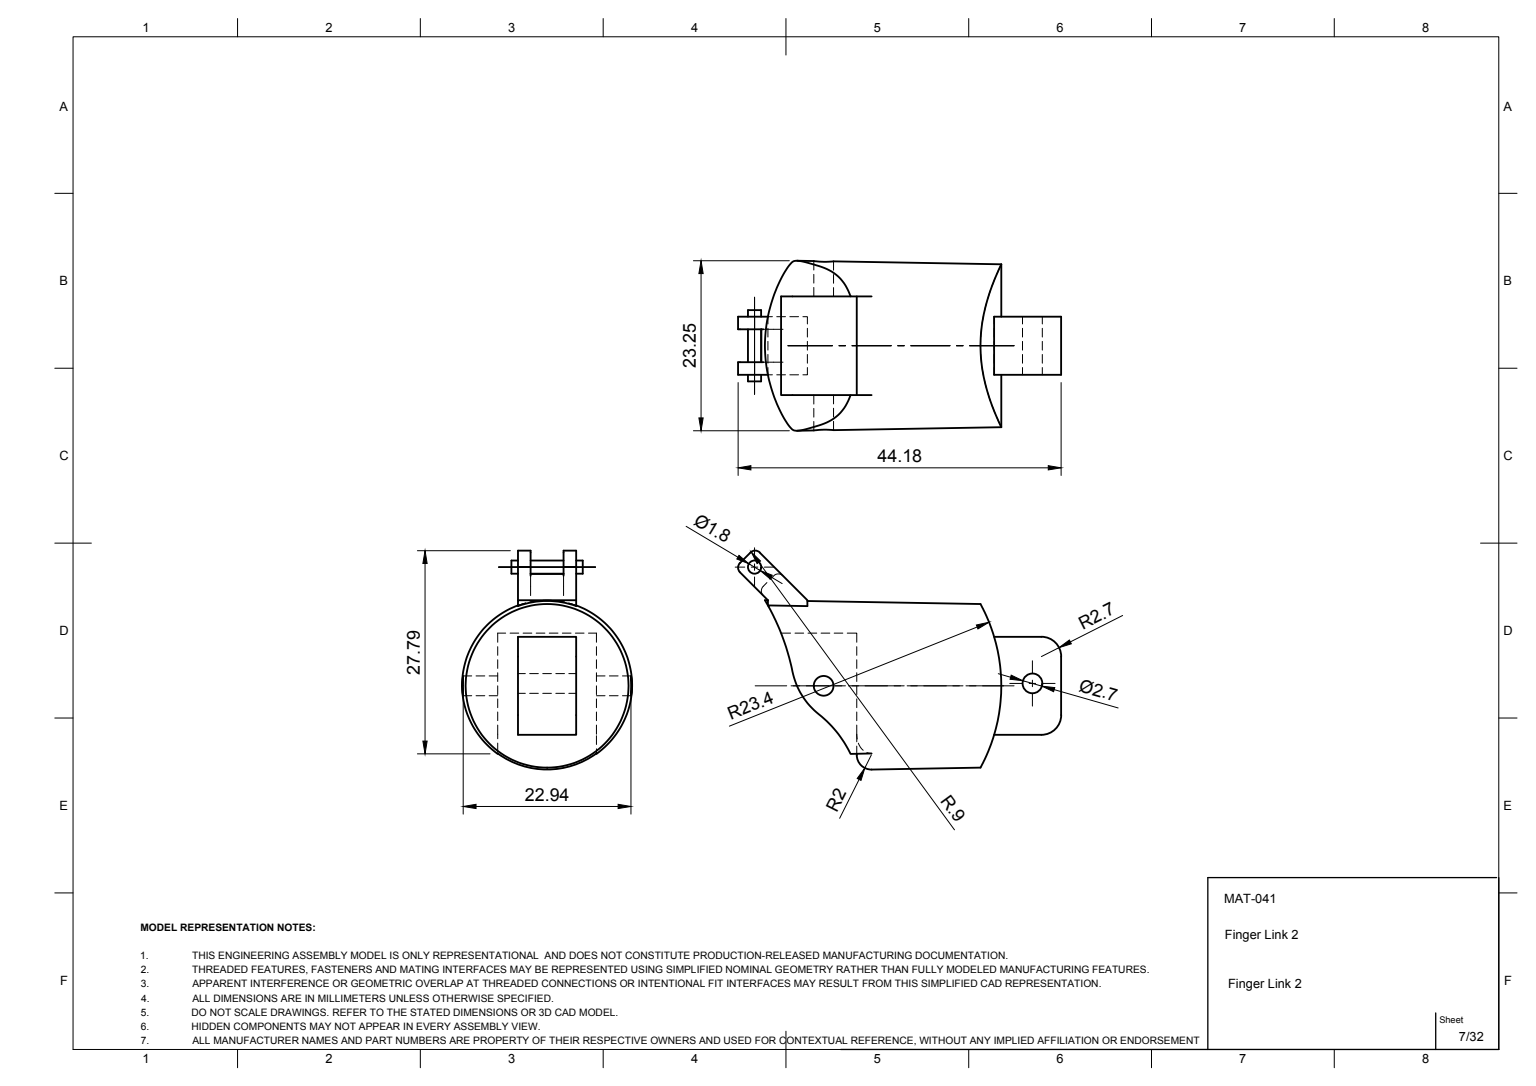
ISO-10303-21;
HEADER;
/* Generated by software containing ST-Developer
 * from STEP Tools, Inc. (www.steptools.com) 
 */

FILE_DESCRIPTION(
/* description */ ('STEP AP214'),
/* implementation_level */ '2;1');

FILE_NAME(
/* name */ 'Finger Link 2.step',
/* time_stamp */ '2026-11-14T21:57:47-08:00',
/* author */ (''),
/* organization */ (''),
/* preprocessor_version */ 'ST-DEVELOPER v20.2',
/* originating_system */ 'Autodesk Translation Framework v15.17.0.0',
/* authorisation */ '');

FILE_SCHEMA (('AUTOMOTIVE_DESIGN { 1 0 10303 214 3 1 1 }'));
ENDSEC;

DATA;
#10=MECHANICAL_DESIGN_GEOMETRIC_PRESENTATION_REPRESENTATION('',(#250),#13199);
#119=CONICAL_SURFACE('',#7291,11.7,0.0174532925199433);
#120=CONICAL_SURFACE('',#7299,11.7,0.0174532925199433);
#141=B_SPLINE_CURVE_WITH_KNOTS('',3,(#10617,#10618,#10619,#10620,#10621,
#10622,#10623,#10624,#10625,#10626,#10627,#10628,#10629,#10630,#10631,#10632,
#10633,#10634),.UNSPECIFIED.,.F.,.F.,(4,2,2,2,2,2,2,2,4),(1.0177645095144,
1.06859347183877,1.11942243416314,1.17022390747156,1.22102538077998,1.27203011389648,
1.32303484701297,1.37402558782589,1.42501632863882),.UNSPECIFIED.);
#142=B_SPLINE_CURVE_WITH_KNOTS('',3,(#10635,#10636,#10637,#10638,#10639,
#10640,#10641,#10642,#10643,#10644,#10645,#10646,#10647,#10648,#10649,#10650,
#10651,#10652,#10653),.UNSPECIFIED.,.F.,.F.,(4,2,2,2,3,2,2,2,4),(0.610512690389992,
0.661503431202914,0.712494172015835,0.763498905132329,0.814503638248823,
0.865305111557246,0.916106584865669,0.966935547190036,1.0177645095144),
 .UNSPECIFIED.);
#143=B_SPLINE_CURVE_WITH_KNOTS('',3,(#10657,#10658,#10659,#10660,#10661,
#10662,#10663,#10664,#10665,#10666,#10667,#10668,#10669,#10670,#10671,#10672,
#10673,#10674),.UNSPECIFIED.,.F.,.F.,(4,2,2,2,2,2,2,2,4),(-0.610512690389992,
-0.55952194957707,-0.508531208764149,-0.457526475647655,-0.406521742531161,
-0.355720269222738,-0.304918795914315,-0.254089833589948,-0.203260871265581),
 .UNSPECIFIED.);
#144=B_SPLINE_CURVE_WITH_KNOTS('',3,(#10678,#10679,#10680,#10681,#10682,
#10683,#10684,#10685,#10686,#10687,#10688,#10689,#10690,#10691,#10692,#10693,
#10694,#10695,#10696),.UNSPECIFIED.,.F.,.F.,(4,2,2,2,3,2,2,2,4),(-0.203260871265581,
-0.152431908941213,-0.101602946616846,-0.0508014733084231,0.,0.0510047331164938,
0.102009466232988,0.153000207045909,0.203990947858831),.UNSPECIFIED.);
#145=B_SPLINE_CURVE_WITH_KNOTS('',3,(#10702,#10703,#10704,#10705),
 .UNSPECIFIED.,.F.,.F.,(4,4),(0.0320334028505474,0.0349204253098787),
 .UNSPECIFIED.);
#146=B_SPLINE_CURVE_WITH_KNOTS('',3,(#10707,#10708,#10709,#10710,#10711,
#10712,#10713,#10714,#10715,#10716),.UNSPECIFIED.,.F.,.F.,(4,2,2,2,4),(1.8422488924149,
2.04440794331246,2.28720862023162,2.53000929715077,2.64124356821964),
 .UNSPECIFIED.);
#147=B_SPLINE_CURVE_WITH_KNOTS('',3,(#10718,#10719,#10720,#10721,#10722,
#10723,#10724,#10725,#10726,#10727),.UNSPECIFIED.,.F.,.F.,(4,2,2,2,4),(6.38658386410106,
6.48595628344589,6.66853921041904,6.85112213739218,7.0623660754825),
 .UNSPECIFIED.);
#148=B_SPLINE_CURVE_WITH_KNOTS('',3,(#10729,#10730,#10731,#10732,#10733,
#10734,#10735,#10736,#10737,#10738),.UNSPECIFIED.,.F.,.F.,(4,2,2,2,4),(3.96444278282234,
4.01597597737689,4.46288213733859,4.92120866579123,5.18441802586752),
 .UNSPECIFIED.);
#149=B_SPLINE_CURVE_WITH_KNOTS('',3,(#10740,#10741,#10742,#10743,#10744,
#10745,#10746),.UNSPECIFIED.,.F.,.F.,(4,3,4),(0.0201480402418329,0.0228906128443418,
0.0255489715004856),.UNSPECIFIED.);
#150=B_SPLINE_CURVE_WITH_KNOTS('',3,(#10752,#10753,#10754,#10755,#10756,
#10757,#10758,#10759,#10760,#10761,#10762,#10763,#10764,#10765,#10766,#10767,
#10768,#10769,#10770,#10771,#10772,#10773),.UNSPECIFIED.,.F.,.F.,(4,2,2,
2,2,2,2,2,2,2,4),(3.42549582701687,3.63995923491168,3.8544226428065,4.28334945859613,
4.71079343465883,5.13823741072153,5.56568618497645,5.99313495923137,6.42206330663255,
6.63652748033314,6.85099165403373),.UNSPECIFIED.);
#151=B_SPLINE_CURVE_WITH_KNOTS('',3,(#10774,#10775,#10776,#10777,#10778,
#10779,#10780,#10781,#10782,#10783,#10784,#10785,#10786,#10787,#10788,#10789,
#10790,#10791,#10792,#10793,#10794,#10795),.UNSPECIFIED.,.F.,.F.,(4,2,2,
2,2,2,2,2,2,2,4),(0.,0.21446417370059,0.428928347401181,0.857856694802362,
1.28530546905728,1.7127542433122,2.1401982193749,2.5676421954376,2.99656901122723,
3.21103241912205,3.42549582701687),.UNSPECIFIED.);
#152=B_SPLINE_CURVE_WITH_KNOTS('',3,(#10799,#10800,#10801,#10802,#10803,
#10804,#10805),.UNSPECIFIED.,.F.,.F.,(4,3,4),(0.0202322541917222,0.0228906128474993,
0.0256331854496299),.UNSPECIFIED.);
#153=B_SPLINE_CURVE_WITH_KNOTS('',3,(#10807,#10808,#10809,#10810,#10811,
#10812,#10813,#10814,#10815,#10816),.UNSPECIFIED.,.F.,.F.,(4,2,2,2,4),(1.95372160896285,
2.21693096903914,2.67525749749178,3.12216365745348,3.17369685200803),
 .UNSPECIFIED.);
#154=B_SPLINE_CURVE_WITH_KNOTS('',3,(#10818,#10819,#10820,#10821,#10822,
#10823,#10824,#10825,#10826,#10827),.UNSPECIFIED.,.F.,.F.,(4,2,2,2,4),(10.2613045765272,
10.4725485146175,10.6551314415907,10.8377143685638,10.9370867879086),
 .UNSPECIFIED.);
#155=B_SPLINE_CURVE_WITH_KNOTS('',3,(#10829,#10830,#10831,#10832,#10833,
#10834,#10835,#10836,#10837,#10838),.UNSPECIFIED.,.F.,.F.,(4,2,2,2,4),(4.03342707380782,
4.14466134487669,4.38746202179585,4.630262698715,4.83242174961257),
 .UNSPECIFIED.);
#156=B_SPLINE_CURVE_WITH_KNOTS('',3,(#10839,#10840,#10841,#10842),
 .UNSPECIFIED.,.F.,.F.,(4,4),(0.0108996070094278,0.0137866294584668),
 .UNSPECIFIED.);
#157=B_SPLINE_CURVE_WITH_KNOTS('',3,(#10848,#10849,#10850,#10851,#10852,
#10853,#10854,#10855,#10856,#10857),.UNSPECIFIED.,.F.,.F.,(4,2,2,2,4),(-3.96444278282234,
-3.79252289739604,-3.56906981741519,-3.34561673743433,-3.17369685200803),
 .UNSPECIFIED.);
#158=B_SPLINE_CURVE_WITH_KNOTS('',3,(#10897,#10898,#10899,#10900,#10901,
#10902,#10903,#10904,#10905,#10906,#10907,#10908,#10909),.UNSPECIFIED.,
 .F.,.F.,(4,2,2,2,3,4),(-0.346533453564935,-0.234184438198016,-0.144253134532049,
-0.0681159640541859,0.,0.00346167201765239),.UNSPECIFIED.);
#159=B_SPLINE_CURVE_WITH_KNOTS('',3,(#10914,#10915,#10916,#10917,#10918,
#10919,#10920,#10921,#10922,#10923,#10924,#10925,#10926),.UNSPECIFIED.,
 .F.,.F.,(4,3,2,2,2,4),(-0.003464253118063,0.,0.0681159640541862,0.14425313453205,
0.234184438198017,0.346533453564935),.UNSPECIFIED.);
#214=SHAPE_REPRESENTATION_RELATIONSHIP('SRR','None',#13282,#232);
#232=ADVANCED_BREP_SHAPE_REPRESENTATION('',(#268),#13178);
#250=STYLED_ITEM('',(#13409),#268);
#268=MANIFOLD_SOLID_BREP('Body1',#6845);
#301=FACE_BOUND('',#2318,.T.);
#302=FACE_BOUND('',#2319,.T.);
#303=FACE_BOUND('',#2324,.T.);
#304=FACE_BOUND('',#2327,.T.);
#305=FACE_BOUND('',#2329,.T.);
#306=FACE_BOUND('',#2333,.T.);
#307=FACE_BOUND('',#2336,.T.);
#308=FACE_BOUND('',#2342,.T.);
#309=FACE_BOUND('',#2344,.T.);
#310=FACE_BOUND('',#2355,.T.);
#311=FACE_BOUND('',#2358,.T.);
#441=PLANE('',#7298);
#442=PLANE('',#7304);
#443=PLANE('',#7306);
#444=PLANE('',#7309);
#445=PLANE('',#7312);
#446=PLANE('',#7313);
#447=PLANE('',#7314);
#448=PLANE('',#7317);
#449=PLANE('',#7318);
#450=PLANE('',#7321);
#451=PLANE('',#7322);
#452=PLANE('',#7323);
#453=PLANE('',#7324);
#454=PLANE('',#7325);
#455=PLANE('',#7330);
#456=PLANE('',#7335);
#457=PLANE('',#7336);
#458=PLANE('',#7343);
#459=PLANE('',#7344);
#460=PLANE('',#7347);
#461=PLANE('',#7348);
#462=PLANE('',#7351);
#734=LINE('',#10591,#1252);
#735=LINE('',#10597,#1253);
#736=LINE('',#10603,#1254);
#737=LINE('',#10609,#1255);
#738=LINE('',#10615,#1256);
#739=LINE('',#10676,#1257);
#740=LINE('',#10750,#1258);
#741=LINE('',#10847,#1259);
#742=LINE('',#10859,#1260);
#743=LINE('',#10862,#1261);
#744=LINE('',#10866,#1262);
#745=LINE('',#10868,#1263);
#746=LINE('',#10870,#1264);
#747=LINE('',#10871,#1265);
#748=LINE('',#10877,#1266);
#749=LINE('',#10881,#1267);
#750=LINE('',#10888,#1268);
#751=LINE('',#10890,#1269);
#752=LINE('',#10891,#1270);
#753=LINE('',#10896,#1271);
#754=LINE('',#10927,#1272);
#755=LINE('',#10931,#1273);
#756=LINE('',#10933,#1274);
#757=LINE('',#10934,#1275);
#758=LINE('',#10938,#1276);
#759=LINE('',#10942,#1277);
#760=LINE('',#10943,#1278);
#761=LINE('',#10945,#1279);
#762=LINE('',#10949,#1280);
#763=LINE('',#10950,#1281);
#764=LINE('',#10953,#1282);
#765=LINE('',#10957,#1283);
#766=LINE('',#10960,#1284);
#767=LINE('',#10962,#1285);
#768=LINE('',#10964,#1286);
#769=LINE('',#10966,#1287);
#770=LINE('',#10967,#1288);
#771=LINE('',#10971,#1289);
#772=LINE('',#10973,#1290);
#773=LINE('',#10975,#1291);
#774=LINE('',#10976,#1292);
#775=LINE('',#10977,#1293);
#776=LINE('',#10981,#1294);
#777=LINE('',#10982,#1295);
#778=LINE('',#10983,#1296);
#779=LINE('',#10987,#1297);
#780=LINE('',#10989,#1298);
#781=LINE('',#10991,#1299);
#782=LINE('',#10992,#1300);
#783=LINE('',#11014,#1301);
#784=LINE('',#11016,#1302);
#785=LINE('',#11018,#1303);
#786=LINE('',#11019,#1304);
#787=LINE('',#11022,#1305);
#788=LINE('',#11026,#1306);
#789=LINE('',#11029,#1307);
#790=LINE('',#11030,#1308);
#791=LINE('',#11034,#1309);
#792=LINE('',#11037,#1310);
#793=LINE('',#11041,#1311);
#794=LINE('',#11043,#1312);
#1252=VECTOR('',#8387,1.35);
#1253=VECTOR('',#8394,0.900000000000001);
#1254=VECTOR('',#8401,0.900000000000001);
#1255=VECTOR('',#8408,0.900000000000001);
#1256=VECTOR('',#8415,1.35);
#1257=VECTOR('',#8418,1.35);
#1258=VECTOR('',#8427,11.7);
#1259=VECTOR('',#8434,1000.);
#1260=VECTOR('',#8435,1000.);
#1261=VECTOR('',#8438,1000.);
#1262=VECTOR('',#8441,1000.);
#1263=VECTOR('',#8442,1000.);
#1264=VECTOR('',#8443,1000.);
#1265=VECTOR('',#8444,1000.);
#1266=VECTOR('',#8451,1000.);
#1267=VECTOR('',#8454,1000.);
#1268=VECTOR('',#8461,1000.);
#1269=VECTOR('',#8462,1000.);
#1270=VECTOR('',#8463,1000.);
#1271=VECTOR('',#8470,1000.);
#1272=VECTOR('',#8477,1000.);
#1273=VECTOR('',#8482,1000.);
#1274=VECTOR('',#8483,1000.);
#1275=VECTOR('',#8484,1000.);
#1276=VECTOR('',#8487,1000.);
#1277=VECTOR('',#8490,1000.);
#1278=VECTOR('',#8491,1000.);
#1279=VECTOR('',#8492,1000.);
#1280=VECTOR('',#8497,1000.);
#1281=VECTOR('',#8498,1000.);
#1282=VECTOR('',#8501,1000.);
#1283=VECTOR('',#8506,1000.);
#1284=VECTOR('',#8509,1000.);
#1285=VECTOR('',#8510,1000.);
#1286=VECTOR('',#8511,1000.);
#1287=VECTOR('',#8512,1000.);
#1288=VECTOR('',#8513,1000.);
#1289=VECTOR('',#8516,1000.);
#1290=VECTOR('',#8517,1000.);
#1291=VECTOR('',#8518,1000.);
#1292=VECTOR('',#8519,1000.);
#1293=VECTOR('',#8520,1000.);
#1294=VECTOR('',#8523,1000.);
#1295=VECTOR('',#8524,1000.);
#1296=VECTOR('',#8525,1000.);
#1297=VECTOR('',#8528,1000.);
#1298=VECTOR('',#8529,1000.);
#1299=VECTOR('',#8530,1000.);
#1300=VECTOR('',#8531,1000.);
#1301=VECTOR('',#8570,1000.);
#1302=VECTOR('',#8571,1000.);
#1303=VECTOR('',#8572,1000.);
#1304=VECTOR('',#8573,1000.);
#1305=VECTOR('',#8576,1000.);
#1306=VECTOR('',#8581,1000.);
#1307=VECTOR('',#8584,1000.);
#1308=VECTOR('',#8585,1000.);
#1309=VECTOR('',#8590,1000.);
#1310=VECTOR('',#8595,1000.);
#1311=VECTOR('',#8602,1000.);
#1312=VECTOR('',#8605,1000.);
#1685=CYLINDRICAL_SURFACE('',#7275,1.35);
#1686=CYLINDRICAL_SURFACE('',#7278,0.900000000000001);
#1687=CYLINDRICAL_SURFACE('',#7281,0.900000000000001);
#1688=CYLINDRICAL_SURFACE('',#7284,0.900000000000001);
#1689=CYLINDRICAL_SURFACE('',#7287,1.35);
#1690=CYLINDRICAL_SURFACE('',#7289,1.35);
#1691=CYLINDRICAL_SURFACE('',#7295,31.5);
#1692=CYLINDRICAL_SURFACE('',#7301,23.4);
#1693=CYLINDRICAL_SURFACE('',#7337,0.9);
#1694=CYLINDRICAL_SURFACE('',#7338,0.9);
#1695=CYLINDRICAL_SURFACE('',#7339,0.9);
#1696=CYLINDRICAL_SURFACE('',#7340,0.9);
#1697=CYLINDRICAL_SURFACE('',#7341,0.9);
#1698=CYLINDRICAL_SURFACE('',#7342,0.9);
#1699=CYLINDRICAL_SURFACE('',#7352,2.7);
#1700=CYLINDRICAL_SURFACE('',#7353,2.7);
#1701=CYLINDRICAL_SURFACE('',#7354,15.4750964764976);
#1702=CYLINDRICAL_SURFACE('',#7355,15.4750964764976);
#1703=CYLINDRICAL_SURFACE('',#7356,10.);
#1704=CYLINDRICAL_SURFACE('',#7357,10.);
#1903=FACE_OUTER_BOUND('',#2311,.T.);
#1904=FACE_OUTER_BOUND('',#2312,.T.);
#1905=FACE_OUTER_BOUND('',#2313,.T.);
#1906=FACE_OUTER_BOUND('',#2314,.T.);
#1907=FACE_OUTER_BOUND('',#2315,.T.);
#1908=FACE_OUTER_BOUND('',#2316,.T.);
#1909=FACE_OUTER_BOUND('',#2317,.T.);
#1910=FACE_OUTER_BOUND('',#2320,.T.);
#1911=FACE_OUTER_BOUND('',#2321,.T.);
#1912=FACE_OUTER_BOUND('',#2322,.T.);
#1913=FACE_OUTER_BOUND('',#2323,.T.);
#1914=FACE_OUTER_BOUND('',#2325,.T.);
#1915=FACE_OUTER_BOUND('',#2326,.T.);
#1916=FACE_OUTER_BOUND('',#2328,.T.);
#1917=FACE_OUTER_BOUND('',#2330,.T.);
#1918=FACE_OUTER_BOUND('',#2331,.T.);
#1919=FACE_OUTER_BOUND('',#2332,.T.);
#1920=FACE_OUTER_BOUND('',#2334,.T.);
#1921=FACE_OUTER_BOUND('',#2335,.T.);
#1922=FACE_OUTER_BOUND('',#2337,.T.);
#1923=FACE_OUTER_BOUND('',#2338,.T.);
#1924=FACE_OUTER_BOUND('',#2339,.T.);
#1925=FACE_OUTER_BOUND('',#2340,.T.);
#1926=FACE_OUTER_BOUND('',#2341,.T.);
#1927=FACE_OUTER_BOUND('',#2343,.T.);
#1928=FACE_OUTER_BOUND('',#2345,.T.);
#1929=FACE_OUTER_BOUND('',#2346,.T.);
#1930=FACE_OUTER_BOUND('',#2347,.T.);
#1931=FACE_OUTER_BOUND('',#2348,.T.);
#1932=FACE_OUTER_BOUND('',#2349,.T.);
#1933=FACE_OUTER_BOUND('',#2350,.T.);
#1934=FACE_OUTER_BOUND('',#2351,.T.);
#1935=FACE_OUTER_BOUND('',#2352,.T.);
#1936=FACE_OUTER_BOUND('',#2353,.T.);
#1937=FACE_OUTER_BOUND('',#2354,.T.);
#1938=FACE_OUTER_BOUND('',#2356,.T.);
#1939=FACE_OUTER_BOUND('',#2357,.T.);
#1940=FACE_OUTER_BOUND('',#2359,.T.);
#1941=FACE_OUTER_BOUND('',#2360,.T.);
#1942=FACE_OUTER_BOUND('',#2361,.T.);
#1943=FACE_OUTER_BOUND('',#2362,.T.);
#1944=FACE_OUTER_BOUND('',#2363,.T.);
#1945=FACE_OUTER_BOUND('',#2364,.T.);
#1946=FACE_OUTER_BOUND('',#2365,.T.);
#1947=FACE_OUTER_BOUND('',#2366,.T.);
#2311=EDGE_LOOP('',(#5048,#5049,#5050,#5051));
#2312=EDGE_LOOP('',(#5052,#5053,#5054,#5055));
#2313=EDGE_LOOP('',(#5056,#5057,#5058,#5059));
#2314=EDGE_LOOP('',(#5060,#5061,#5062,#5063));
#2315=EDGE_LOOP('',(#5064,#5065,#5066,#5067,#5068));
#2316=EDGE_LOOP('',(#5069,#5070,#5071,#5072,#5073));
#2317=EDGE_LOOP('',(#5074,#5075,#5076,#5077,#5078,#5079,#5080,#5081,#5082,
#5083,#5084,#5085,#5086,#5087,#5088,#5089,#5090));
#2318=EDGE_LOOP('',(#5091,#5092));
#2319=EDGE_LOOP('',(#5093,#5094));
#2320=EDGE_LOOP('',(#5095,#5096,#5097,#5098,#5099,#5100,#5101,#5102));
#2321=EDGE_LOOP('',(#5103,#5104,#5105,#5106));
#2322=EDGE_LOOP('',(#5107,#5108));
#2323=EDGE_LOOP('',(#5109,#5110));
#2324=EDGE_LOOP('',(#5111,#5112,#5113,#5114));
#2325=EDGE_LOOP('',(#5115,#5116,#5117,#5118));
#2326=EDGE_LOOP('',(#5119,#5120,#5121,#5122,#5123,#5124,#5125));
#2327=EDGE_LOOP('',(#5126));
#2328=EDGE_LOOP('',(#5127,#5128,#5129,#5130,#5131,#5132,#5133));
#2329=EDGE_LOOP('',(#5134));
#2330=EDGE_LOOP('',(#5135,#5136,#5137,#5138));
#2331=EDGE_LOOP('',(#5139,#5140,#5141,#5142));
#2332=EDGE_LOOP('',(#5143,#5144,#5145,#5146,#5147,#5148,#5149,#5150));
#2333=EDGE_LOOP('',(#5151));
#2334=EDGE_LOOP('',(#5152,#5153,#5154,#5155,#5156));
#2335=EDGE_LOOP('',(#5157,#5158,#5159,#5160,#5161,#5162,#5163,#5164));
#2336=EDGE_LOOP('',(#5165));
#2337=EDGE_LOOP('',(#5166,#5167,#5168,#5169,#5170,#5171,#5172,#5173));
#2338=EDGE_LOOP('',(#5174,#5175,#5176,#5177,#5178,#5179,#5180,#5181));
#2339=EDGE_LOOP('',(#5182,#5183,#5184,#5185));
#2340=EDGE_LOOP('',(#5186,#5187,#5188,#5189));
#2341=EDGE_LOOP('',(#5190,#5191,#5192,#5193,#5194,#5195,#5196,#5197));
#2342=EDGE_LOOP('',(#5198));
#2343=EDGE_LOOP('',(#5199,#5200,#5201,#5202,#5203,#5204,#5205,#5206));
#2344=EDGE_LOOP('',(#5207));
#2345=EDGE_LOOP('',(#5208));
#2346=EDGE_LOOP('',(#5209));
#2347=EDGE_LOOP('',(#5210,#5211,#5212,#5213));
#2348=EDGE_LOOP('',(#5214,#5215,#5216,#5217));
#2349=EDGE_LOOP('',(#5218,#5219,#5220,#5221));
#2350=EDGE_LOOP('',(#5222,#5223,#5224,#5225));
#2351=EDGE_LOOP('',(#5226,#5227,#5228,#5229));
#2352=EDGE_LOOP('',(#5230,#5231,#5232,#5233));
#2353=EDGE_LOOP('',(#5234,#5235,#5236,#5237));
#2354=EDGE_LOOP('',(#5238,#5239,#5240,#5241,#5242,#5243));
#2355=EDGE_LOOP('',(#5244));
#2356=EDGE_LOOP('',(#5245,#5246,#5247,#5248));
#2357=EDGE_LOOP('',(#5249,#5250,#5251,#5252,#5253,#5254));
#2358=EDGE_LOOP('',(#5255));
#2359=EDGE_LOOP('',(#5256,#5257,#5258,#5259));
#2360=EDGE_LOOP('',(#5260,#5261,#5262,#5263));
#2361=EDGE_LOOP('',(#5264,#5265,#5266,#5267));
#2362=EDGE_LOOP('',(#5268,#5269,#5270));
#2363=EDGE_LOOP('',(#5271,#5272,#5273));
#2364=EDGE_LOOP('',(#5274,#5275,#5276,#5277));
#2365=EDGE_LOOP('',(#5278,#5279,#5280,#5281));
#2366=EDGE_LOOP('',(#5282,#5283,#5284,#5285));
#2779=CIRCLE('',#7276,1.35);
#2780=CIRCLE('',#7277,1.35);
#2781=CIRCLE('',#7279,0.900000000000001);
#2782=CIRCLE('',#7280,0.900000000000001);
#2783=CIRCLE('',#7282,0.900000000000001);
#2784=CIRCLE('',#7283,0.900000000000001);
#2785=CIRCLE('',#7285,0.900000000000001);
#2786=CIRCLE('',#7286,0.900000000000001);
#2787=CIRCLE('',#7288,1.35);
#2788=CIRCLE('',#7290,1.35);
#2789=CIRCLE('',#7292,11.4453313393709);
#2790=CIRCLE('',#7293,11.5986607340431);
#2791=CIRCLE('',#7294,11.5986607340431);
#2792=CIRCLE('',#7296,31.5);
#2793=CIRCLE('',#7297,31.5);
#2794=CIRCLE('',#7300,11.6929180846555);
#2795=CIRCLE('',#7302,23.4);
#2796=CIRCLE('',#7303,23.4);
#2797=CIRCLE('',#7305,9.44563594905814);
#2798=CIRCLE('',#7307,15.4750964764976);
#2799=CIRCLE('',#7308,10.);
#2800=CIRCLE('',#7310,10.);
#2801=CIRCLE('',#7311,15.4750964764976);
#2802=CIRCLE('',#7315,0.9);
#2803=CIRCLE('',#7316,0.9);
#2804=CIRCLE('',#7319,0.9);
#2805=CIRCLE('',#7320,0.9);
#2806=CIRCLE('',#7326,0.9);
#2807=CIRCLE('',#7327,0.9);
#2808=CIRCLE('',#7328,0.9);
#2809=CIRCLE('',#7329,0.9);
#2810=CIRCLE('',#7331,0.9);
#2811=CIRCLE('',#7332,0.9);
#2812=CIRCLE('',#7333,0.9);
#2813=CIRCLE('',#7334,0.9);
#2814=CIRCLE('',#7345,2.7);
#2815=CIRCLE('',#7346,2.7);
#2816=CIRCLE('',#7349,2.7);
#2817=CIRCLE('',#7350,2.7);
#3151=VERTEX_POINT('',#10588);
#3152=VERTEX_POINT('',#10590);
#3153=VERTEX_POINT('',#10594);
#3154=VERTEX_POINT('',#10596);
#3155=VERTEX_POINT('',#10600);
#3156=VERTEX_POINT('',#10602);
#3157=VERTEX_POINT('',#10606);
#3158=VERTEX_POINT('',#10608);
#3159=VERTEX_POINT('',#10612);
#3160=VERTEX_POINT('',#10614);
#3161=VERTEX_POINT('',#10616);
#3162=VERTEX_POINT('',#10655);
#3163=VERTEX_POINT('',#10656);
#3164=VERTEX_POINT('',#10675);
#3165=VERTEX_POINT('',#10698);
#3166=VERTEX_POINT('',#10699);
#3167=VERTEX_POINT('',#10701);
#3168=VERTEX_POINT('',#10706);
#3169=VERTEX_POINT('',#10717);
#3170=VERTEX_POINT('',#10728);
#3171=VERTEX_POINT('',#10739);
#3172=VERTEX_POINT('',#10747);
#3173=VERTEX_POINT('',#10749);
#3174=VERTEX_POINT('',#10751);
#3175=VERTEX_POINT('',#10796);
#3176=VERTEX_POINT('',#10798);
#3177=VERTEX_POINT('',#10806);
#3178=VERTEX_POINT('',#10817);
#3179=VERTEX_POINT('',#10828);
#3180=VERTEX_POINT('',#10844);
#3181=VERTEX_POINT('',#10845);
#3182=VERTEX_POINT('',#10858);
#3183=VERTEX_POINT('',#10860);
#3184=VERTEX_POINT('',#10864);
#3185=VERTEX_POINT('',#10865);
#3186=VERTEX_POINT('',#10867);
#3187=VERTEX_POINT('',#10869);
#3188=VERTEX_POINT('',#10875);
#3189=VERTEX_POINT('',#10876);
#3190=VERTEX_POINT('',#10878);
#3191=VERTEX_POINT('',#10880);
#3192=VERTEX_POINT('',#10884);
#3193=VERTEX_POINT('',#10885);
#3194=VERTEX_POINT('',#10887);
#3195=VERTEX_POINT('',#10889);
#3196=VERTEX_POINT('',#10893);
#3197=VERTEX_POINT('',#10911);
#3198=VERTEX_POINT('',#10930);
#3199=VERTEX_POINT('',#10932);
#3200=VERTEX_POINT('',#10936);
#3201=VERTEX_POINT('',#10937);
#3202=VERTEX_POINT('',#10939);
#3203=VERTEX_POINT('',#10941);
#3204=VERTEX_POINT('',#10944);
#3205=VERTEX_POINT('',#10948);
#3206=VERTEX_POINT('',#10952);
#3207=VERTEX_POINT('',#10955);
#3208=VERTEX_POINT('',#10959);
#3209=VERTEX_POINT('',#10961);
#3210=VERTEX_POINT('',#10963);
#3211=VERTEX_POINT('',#10965);
#3212=VERTEX_POINT('',#10969);
#3213=VERTEX_POINT('',#10970);
#3214=VERTEX_POINT('',#10972);
#3215=VERTEX_POINT('',#10974);
#3216=VERTEX_POINT('',#10979);
#3217=VERTEX_POINT('',#10980);
#3218=VERTEX_POINT('',#10985);
#3219=VERTEX_POINT('',#10986);
#3220=VERTEX_POINT('',#10988);
#3221=VERTEX_POINT('',#10990);
#3222=VERTEX_POINT('',#11012);
#3223=VERTEX_POINT('',#11013);
#3224=VERTEX_POINT('',#11015);
#3225=VERTEX_POINT('',#11017);
#3226=VERTEX_POINT('',#11021);
#3227=VERTEX_POINT('',#11024);
#3228=VERTEX_POINT('',#11028);
#3229=VERTEX_POINT('',#11033);
#3861=EDGE_CURVE('',#3151,#3151,#2779,.T.);
#3862=EDGE_CURVE('',#3151,#3152,#734,.T.);
#3863=EDGE_CURVE('',#3152,#3152,#2780,.T.);
#3864=EDGE_CURVE('',#3153,#3153,#2781,.T.);
#3865=EDGE_CURVE('',#3153,#3154,#735,.T.);
#3866=EDGE_CURVE('',#3154,#3154,#2782,.T.);
#3867=EDGE_CURVE('',#3155,#3155,#2783,.T.);
#3868=EDGE_CURVE('',#3155,#3156,#736,.T.);
#3869=EDGE_CURVE('',#3156,#3156,#2784,.T.);
#3870=EDGE_CURVE('',#3157,#3157,#2785,.T.);
#3871=EDGE_CURVE('',#3157,#3158,#737,.T.);
#3872=EDGE_CURVE('',#3158,#3158,#2786,.T.);
#3873=EDGE_CURVE('',#3159,#3159,#2787,.T.);
#3874=EDGE_CURVE('',#3159,#3160,#738,.T.);
#3875=EDGE_CURVE('',#3160,#3161,#141,.T.);
#3876=EDGE_CURVE('',#3161,#3160,#142,.T.);
#3877=EDGE_CURVE('',#3162,#3163,#143,.T.);
#3878=EDGE_CURVE('',#3163,#3164,#739,.T.);
#3879=EDGE_CURVE('',#3164,#3164,#2788,.T.);
#3880=EDGE_CURVE('',#3163,#3162,#144,.T.);
#3881=EDGE_CURVE('',#3165,#3166,#2789,.T.);
#3882=EDGE_CURVE('',#3167,#3166,#145,.T.);
#3883=EDGE_CURVE('',#3168,#3167,#146,.T.);
#3884=EDGE_CURVE('',#3168,#3169,#147,.T.);
#3885=EDGE_CURVE('',#3170,#3169,#148,.T.);
#3886=EDGE_CURVE('',#3170,#3171,#149,.T.);
#3887=EDGE_CURVE('',#3171,#3172,#2790,.T.);
#3888=EDGE_CURVE('',#3172,#3173,#740,.T.);
#3889=EDGE_CURVE('',#3173,#3174,#150,.T.);
#3890=EDGE_CURVE('',#3174,#3173,#151,.T.);
#3891=EDGE_CURVE('',#3172,#3175,#2791,.T.);
#3892=EDGE_CURVE('',#3175,#3176,#152,.T.);
#3893=EDGE_CURVE('',#3177,#3176,#153,.T.);
#3894=EDGE_CURVE('',#3177,#3178,#154,.T.);
#3895=EDGE_CURVE('',#3179,#3178,#155,.T.);
#3896=EDGE_CURVE('',#3165,#3179,#156,.T.);
#3897=EDGE_CURVE('',#3180,#3181,#2792,.T.);
#3898=EDGE_CURVE('',#3181,#3177,#741,.T.);
#3899=EDGE_CURVE('',#3176,#3170,#157,.T.);
#3900=EDGE_CURVE('',#3169,#3182,#742,.T.);
#3901=EDGE_CURVE('',#3182,#3183,#2793,.T.);
#3902=EDGE_CURVE('',#3180,#3183,#743,.T.);
#3903=EDGE_CURVE('',#3184,#3185,#744,.T.);
#3904=EDGE_CURVE('',#3185,#3186,#745,.T.);
#3905=EDGE_CURVE('',#3187,#3186,#746,.T.);
#3906=EDGE_CURVE('',#3187,#3184,#747,.T.);
#3907=EDGE_CURVE('',#3176,#3170,#2794,.T.);
#3908=EDGE_CURVE('',#3188,#3189,#748,.T.);
#3909=EDGE_CURVE('',#3190,#3188,#2795,.T.);
#3910=EDGE_CURVE('',#3191,#3190,#749,.T.);
#3911=EDGE_CURVE('',#3189,#3191,#2796,.T.);
#3912=EDGE_CURVE('',#3192,#3193,#2797,.T.);
#3913=EDGE_CURVE('',#3193,#3194,#750,.T.);
#3914=EDGE_CURVE('',#3195,#3194,#751,.T.);
#3915=EDGE_CURVE('',#3192,#3195,#752,.T.);
#3916=EDGE_CURVE('',#3179,#3196,#2798,.T.);
#3917=EDGE_CURVE('',#3196,#3181,#2799,.T.);
#3918=EDGE_CURVE('',#3194,#3180,#753,.T.);
#3919=EDGE_CURVE('',#3193,#3165,#158,.T.);
#3920=EDGE_CURVE('',#3182,#3197,#2800,.T.);
#3921=EDGE_CURVE('',#3197,#3167,#2801,.T.);
#3922=EDGE_CURVE('',#3166,#3192,#159,.T.);
#3923=EDGE_CURVE('',#3183,#3195,#754,.T.);
#3924=EDGE_CURVE('',#3176,#3198,#755,.T.);
#3925=EDGE_CURVE('',#3198,#3199,#756,.T.);
#3926=EDGE_CURVE('',#3170,#3199,#757,.T.);
#3927=EDGE_CURVE('',#3200,#3201,#758,.T.);
#3928=EDGE_CURVE('',#3200,#3202,#2802,.T.);
#3929=EDGE_CURVE('',#3202,#3203,#759,.T.);
#3930=EDGE_CURVE('',#3171,#3203,#760,.T.);
#3931=EDGE_CURVE('',#3204,#3199,#761,.T.);
#3932=EDGE_CURVE('',#3204,#3201,#2803,.T.);
#3933=EDGE_CURVE('',#3203,#3205,#762,.T.);
#3934=EDGE_CURVE('',#3175,#3205,#763,.T.);
#3935=EDGE_CURVE('',#3206,#3205,#764,.T.);
#3936=EDGE_CURVE('',#3206,#3185,#2804,.T.);
#3937=EDGE_CURVE('',#3184,#3207,#2805,.T.);
#3938=EDGE_CURVE('',#3207,#3198,#765,.T.);
#3939=EDGE_CURVE('',#3207,#3208,#766,.T.);
#3940=EDGE_CURVE('',#3208,#3209,#767,.T.);
#3941=EDGE_CURVE('',#3209,#3210,#768,.T.);
#3942=EDGE_CURVE('',#3210,#3211,#769,.T.);
#3943=EDGE_CURVE('',#3211,#3204,#770,.T.);
#3944=EDGE_CURVE('',#3212,#3213,#771,.T.);
#3945=EDGE_CURVE('',#3212,#3214,#772,.T.);
#3946=EDGE_CURVE('',#3215,#3214,#773,.T.);
#3947=EDGE_CURVE('',#3215,#3206,#774,.T.);
#3948=EDGE_CURVE('',#3202,#3213,#775,.T.);
#3949=EDGE_CURVE('',#3216,#3217,#776,.T.);
#3950=EDGE_CURVE('',#3216,#3200,#777,.T.);
#3951=EDGE_CURVE('',#3201,#3217,#778,.T.);
#3952=EDGE_CURVE('',#3218,#3219,#779,.T.);
#3953=EDGE_CURVE('',#3219,#3220,#780,.T.);
#3954=EDGE_CURVE('',#3221,#3220,#781,.T.);
#3955=EDGE_CURVE('',#3221,#3218,#782,.T.);
#3956=EDGE_CURVE('',#3186,#3215,#2806,.T.);
#3957=EDGE_CURVE('',#3214,#3219,#2807,.T.);
#3958=EDGE_CURVE('',#3218,#3209,#2808,.T.);
#3959=EDGE_CURVE('',#3208,#3187,#2809,.T.);
#3960=EDGE_CURVE('',#3213,#3216,#2810,.T.);
#3961=EDGE_CURVE('',#3217,#3211,#2811,.T.);
#3962=EDGE_CURVE('',#3210,#3221,#2812,.T.);
#3963=EDGE_CURVE('',#3220,#3212,#2813,.T.);
#3964=EDGE_CURVE('',#3222,#3223,#783,.T.);
#3965=EDGE_CURVE('',#3223,#3224,#784,.T.);
#3966=EDGE_CURVE('',#3224,#3225,#785,.T.);
#3967=EDGE_CURVE('',#3225,#3222,#786,.T.);
#3968=EDGE_CURVE('',#3188,#3226,#787,.T.);
#3969=EDGE_CURVE('',#3226,#3223,#2814,.T.);
#3970=EDGE_CURVE('',#3222,#3227,#2815,.T.);
#3971=EDGE_CURVE('',#3190,#3227,#788,.T.);
#3972=EDGE_CURVE('',#3189,#3228,#789,.T.);
#3973=EDGE_CURVE('',#3228,#3226,#790,.T.);
#3974=EDGE_CURVE('',#3224,#3228,#2816,.T.);
#3975=EDGE_CURVE('',#3191,#3229,#791,.T.);
#3976=EDGE_CURVE('',#3229,#3225,#2817,.T.);
#3977=EDGE_CURVE('',#3227,#3229,#792,.T.);
#3978=EDGE_CURVE('',#3197,#3168,#793,.T.);
#3979=EDGE_CURVE('',#3178,#3196,#794,.T.);
#5048=ORIENTED_EDGE('',*,*,#3861,.T.);
#5049=ORIENTED_EDGE('',*,*,#3862,.T.);
#5050=ORIENTED_EDGE('',*,*,#3863,.T.);
#5051=ORIENTED_EDGE('',*,*,#3862,.F.);
#5052=ORIENTED_EDGE('',*,*,#3864,.T.);
#5053=ORIENTED_EDGE('',*,*,#3865,.T.);
#5054=ORIENTED_EDGE('',*,*,#3866,.T.);
#5055=ORIENTED_EDGE('',*,*,#3865,.F.);
#5056=ORIENTED_EDGE('',*,*,#3867,.T.);
#5057=ORIENTED_EDGE('',*,*,#3868,.T.);
#5058=ORIENTED_EDGE('',*,*,#3869,.F.);
#5059=ORIENTED_EDGE('',*,*,#3868,.F.);
#5060=ORIENTED_EDGE('',*,*,#3870,.T.);
#5061=ORIENTED_EDGE('',*,*,#3871,.T.);
#5062=ORIENTED_EDGE('',*,*,#3872,.T.);
#5063=ORIENTED_EDGE('',*,*,#3871,.F.);
#5064=ORIENTED_EDGE('',*,*,#3873,.F.);
#5065=ORIENTED_EDGE('',*,*,#3874,.T.);
#5066=ORIENTED_EDGE('',*,*,#3875,.T.);
#5067=ORIENTED_EDGE('',*,*,#3876,.T.);
#5068=ORIENTED_EDGE('',*,*,#3874,.F.);
#5069=ORIENTED_EDGE('',*,*,#3877,.T.);
#5070=ORIENTED_EDGE('',*,*,#3878,.T.);
#5071=ORIENTED_EDGE('',*,*,#3879,.F.);
#5072=ORIENTED_EDGE('',*,*,#3878,.F.);
#5073=ORIENTED_EDGE('',*,*,#3880,.T.);
#5074=ORIENTED_EDGE('',*,*,#3881,.T.);
#5075=ORIENTED_EDGE('',*,*,#3882,.F.);
#5076=ORIENTED_EDGE('',*,*,#3883,.F.);
#5077=ORIENTED_EDGE('',*,*,#3884,.T.);
#5078=ORIENTED_EDGE('',*,*,#3885,.F.);
#5079=ORIENTED_EDGE('',*,*,#3886,.T.);
#5080=ORIENTED_EDGE('',*,*,#3887,.T.);
#5081=ORIENTED_EDGE('',*,*,#3888,.T.);
#5082=ORIENTED_EDGE('',*,*,#3889,.T.);
#5083=ORIENTED_EDGE('',*,*,#3890,.T.);
#5084=ORIENTED_EDGE('',*,*,#3888,.F.);
#5085=ORIENTED_EDGE('',*,*,#3891,.T.);
#5086=ORIENTED_EDGE('',*,*,#3892,.T.);
#5087=ORIENTED_EDGE('',*,*,#3893,.F.);
#5088=ORIENTED_EDGE('',*,*,#3894,.T.);
#5089=ORIENTED_EDGE('',*,*,#3895,.F.);
#5090=ORIENTED_EDGE('',*,*,#3896,.F.);
#5091=ORIENTED_EDGE('',*,*,#3877,.F.);
#5092=ORIENTED_EDGE('',*,*,#3880,.F.);
#5093=ORIENTED_EDGE('',*,*,#3876,.F.);
#5094=ORIENTED_EDGE('',*,*,#3875,.F.);
#5095=ORIENTED_EDGE('',*,*,#3897,.T.);
#5096=ORIENTED_EDGE('',*,*,#3898,.T.);
#5097=ORIENTED_EDGE('',*,*,#3893,.T.);
#5098=ORIENTED_EDGE('',*,*,#3899,.T.);
#5099=ORIENTED_EDGE('',*,*,#3885,.T.);
#5100=ORIENTED_EDGE('',*,*,#3900,.T.);
#5101=ORIENTED_EDGE('',*,*,#3901,.T.);
#5102=ORIENTED_EDGE('',*,*,#3902,.F.);
#5103=ORIENTED_EDGE('',*,*,#3903,.T.);
#5104=ORIENTED_EDGE('',*,*,#3904,.T.);
#5105=ORIENTED_EDGE('',*,*,#3905,.F.);
#5106=ORIENTED_EDGE('',*,*,#3906,.T.);
#5107=ORIENTED_EDGE('',*,*,#3907,.T.);
#5108=ORIENTED_EDGE('',*,*,#3899,.F.);
#5109=ORIENTED_EDGE('',*,*,#3890,.F.);
#5110=ORIENTED_EDGE('',*,*,#3889,.F.);
#5111=ORIENTED_EDGE('',*,*,#3908,.F.);
#5112=ORIENTED_EDGE('',*,*,#3909,.F.);
#5113=ORIENTED_EDGE('',*,*,#3910,.F.);
#5114=ORIENTED_EDGE('',*,*,#3911,.F.);
#5115=ORIENTED_EDGE('',*,*,#3912,.T.);
#5116=ORIENTED_EDGE('',*,*,#3913,.T.);
#5117=ORIENTED_EDGE('',*,*,#3914,.F.);
#5118=ORIENTED_EDGE('',*,*,#3915,.F.);
#5119=ORIENTED_EDGE('',*,*,#3916,.T.);
#5120=ORIENTED_EDGE('',*,*,#3917,.T.);
#5121=ORIENTED_EDGE('',*,*,#3897,.F.);
#5122=ORIENTED_EDGE('',*,*,#3918,.F.);
#5123=ORIENTED_EDGE('',*,*,#3913,.F.);
#5124=ORIENTED_EDGE('',*,*,#3919,.T.);
#5125=ORIENTED_EDGE('',*,*,#3896,.T.);
#5126=ORIENTED_EDGE('',*,*,#3873,.T.);
#5127=ORIENTED_EDGE('',*,*,#3901,.F.);
#5128=ORIENTED_EDGE('',*,*,#3920,.T.);
#5129=ORIENTED_EDGE('',*,*,#3921,.T.);
#5130=ORIENTED_EDGE('',*,*,#3882,.T.);
#5131=ORIENTED_EDGE('',*,*,#3922,.T.);
#5132=ORIENTED_EDGE('',*,*,#3915,.T.);
#5133=ORIENTED_EDGE('',*,*,#3923,.F.);
#5134=ORIENTED_EDGE('',*,*,#3879,.T.);
#5135=ORIENTED_EDGE('',*,*,#3902,.T.);
#5136=ORIENTED_EDGE('',*,*,#3923,.T.);
#5137=ORIENTED_EDGE('',*,*,#3914,.T.);
#5138=ORIENTED_EDGE('',*,*,#3918,.T.);
#5139=ORIENTED_EDGE('',*,*,#3907,.F.);
#5140=ORIENTED_EDGE('',*,*,#3924,.T.);
#5141=ORIENTED_EDGE('',*,*,#3925,.T.);
#5142=ORIENTED_EDGE('',*,*,#3926,.F.);
#5143=ORIENTED_EDGE('',*,*,#3927,.F.);
#5144=ORIENTED_EDGE('',*,*,#3928,.T.);
#5145=ORIENTED_EDGE('',*,*,#3929,.T.);
#5146=ORIENTED_EDGE('',*,*,#3930,.F.);
#5147=ORIENTED_EDGE('',*,*,#3886,.F.);
#5148=ORIENTED_EDGE('',*,*,#3926,.T.);
#5149=ORIENTED_EDGE('',*,*,#3931,.F.);
#5150=ORIENTED_EDGE('',*,*,#3932,.T.);
#5151=ORIENTED_EDGE('',*,*,#3866,.F.);
#5152=ORIENTED_EDGE('',*,*,#3887,.F.);
#5153=ORIENTED_EDGE('',*,*,#3930,.T.);
#5154=ORIENTED_EDGE('',*,*,#3933,.T.);
#5155=ORIENTED_EDGE('',*,*,#3934,.F.);
#5156=ORIENTED_EDGE('',*,*,#3891,.F.);
#5157=ORIENTED_EDGE('',*,*,#3935,.F.);
#5158=ORIENTED_EDGE('',*,*,#3936,.T.);
#5159=ORIENTED_EDGE('',*,*,#3903,.F.);
#5160=ORIENTED_EDGE('',*,*,#3937,.T.);
#5161=ORIENTED_EDGE('',*,*,#3938,.T.);
#5162=ORIENTED_EDGE('',*,*,#3924,.F.);
#5163=ORIENTED_EDGE('',*,*,#3892,.F.);
#5164=ORIENTED_EDGE('',*,*,#3934,.T.);
#5165=ORIENTED_EDGE('',*,*,#3867,.F.);
#5166=ORIENTED_EDGE('',*,*,#3938,.F.);
#5167=ORIENTED_EDGE('',*,*,#3939,.T.);
#5168=ORIENTED_EDGE('',*,*,#3940,.T.);
#5169=ORIENTED_EDGE('',*,*,#3941,.T.);
#5170=ORIENTED_EDGE('',*,*,#3942,.T.);
#5171=ORIENTED_EDGE('',*,*,#3943,.T.);
#5172=ORIENTED_EDGE('',*,*,#3931,.T.);
#5173=ORIENTED_EDGE('',*,*,#3925,.F.);
#5174=ORIENTED_EDGE('',*,*,#3944,.F.);
#5175=ORIENTED_EDGE('',*,*,#3945,.T.);
#5176=ORIENTED_EDGE('',*,*,#3946,.F.);
#5177=ORIENTED_EDGE('',*,*,#3947,.T.);
#5178=ORIENTED_EDGE('',*,*,#3935,.T.);
#5179=ORIENTED_EDGE('',*,*,#3933,.F.);
#5180=ORIENTED_EDGE('',*,*,#3929,.F.);
#5181=ORIENTED_EDGE('',*,*,#3948,.T.);
#5182=ORIENTED_EDGE('',*,*,#3949,.F.);
#5183=ORIENTED_EDGE('',*,*,#3950,.T.);
#5184=ORIENTED_EDGE('',*,*,#3927,.T.);
#5185=ORIENTED_EDGE('',*,*,#3951,.T.);
#5186=ORIENTED_EDGE('',*,*,#3952,.T.);
#5187=ORIENTED_EDGE('',*,*,#3953,.T.);
#5188=ORIENTED_EDGE('',*,*,#3954,.F.);
#5189=ORIENTED_EDGE('',*,*,#3955,.T.);
#5190=ORIENTED_EDGE('',*,*,#3905,.T.);
#5191=ORIENTED_EDGE('',*,*,#3956,.T.);
#5192=ORIENTED_EDGE('',*,*,#3946,.T.);
#5193=ORIENTED_EDGE('',*,*,#3957,.T.);
#5194=ORIENTED_EDGE('',*,*,#3952,.F.);
#5195=ORIENTED_EDGE('',*,*,#3958,.T.);
#5196=ORIENTED_EDGE('',*,*,#3940,.F.);
#5197=ORIENTED_EDGE('',*,*,#3959,.T.);
#5198=ORIENTED_EDGE('',*,*,#3872,.F.);
#5199=ORIENTED_EDGE('',*,*,#3944,.T.);
#5200=ORIENTED_EDGE('',*,*,#3960,.T.);
#5201=ORIENTED_EDGE('',*,*,#3949,.T.);
#5202=ORIENTED_EDGE('',*,*,#3961,.T.);
#5203=ORIENTED_EDGE('',*,*,#3942,.F.);
#5204=ORIENTED_EDGE('',*,*,#3962,.T.);
#5205=ORIENTED_EDGE('',*,*,#3954,.T.);
#5206=ORIENTED_EDGE('',*,*,#3963,.T.);
#5207=ORIENTED_EDGE('',*,*,#3870,.F.);
#5208=ORIENTED_EDGE('',*,*,#3869,.T.);
#5209=ORIENTED_EDGE('',*,*,#3864,.F.);
#5210=ORIENTED_EDGE('',*,*,#3957,.F.);
#5211=ORIENTED_EDGE('',*,*,#3945,.F.);
#5212=ORIENTED_EDGE('',*,*,#3963,.F.);
#5213=ORIENTED_EDGE('',*,*,#3953,.F.);
#5214=ORIENTED_EDGE('',*,*,#3960,.F.);
#5215=ORIENTED_EDGE('',*,*,#3948,.F.);
#5216=ORIENTED_EDGE('',*,*,#3928,.F.);
#5217=ORIENTED_EDGE('',*,*,#3950,.F.);
#5218=ORIENTED_EDGE('',*,*,#3936,.F.);
#5219=ORIENTED_EDGE('',*,*,#3947,.F.);
#5220=ORIENTED_EDGE('',*,*,#3956,.F.);
#5221=ORIENTED_EDGE('',*,*,#3904,.F.);
#5222=ORIENTED_EDGE('',*,*,#3959,.F.);
#5223=ORIENTED_EDGE('',*,*,#3939,.F.);
#5224=ORIENTED_EDGE('',*,*,#3937,.F.);
#5225=ORIENTED_EDGE('',*,*,#3906,.F.);
#5226=ORIENTED_EDGE('',*,*,#3932,.F.);
#5227=ORIENTED_EDGE('',*,*,#3943,.F.);
#5228=ORIENTED_EDGE('',*,*,#3961,.F.);
#5229=ORIENTED_EDGE('',*,*,#3951,.F.);
#5230=ORIENTED_EDGE('',*,*,#3958,.F.);
#5231=ORIENTED_EDGE('',*,*,#3955,.F.);
#5232=ORIENTED_EDGE('',*,*,#3962,.F.);
#5233=ORIENTED_EDGE('',*,*,#3941,.F.);
#5234=ORIENTED_EDGE('',*,*,#3964,.T.);
#5235=ORIENTED_EDGE('',*,*,#3965,.T.);
#5236=ORIENTED_EDGE('',*,*,#3966,.T.);
#5237=ORIENTED_EDGE('',*,*,#3967,.T.);
#5238=ORIENTED_EDGE('',*,*,#3968,.T.);
#5239=ORIENTED_EDGE('',*,*,#3969,.T.);
#5240=ORIENTED_EDGE('',*,*,#3964,.F.);
#5241=ORIENTED_EDGE('',*,*,#3970,.T.);
#5242=ORIENTED_EDGE('',*,*,#3971,.F.);
#5243=ORIENTED_EDGE('',*,*,#3909,.T.);
#5244=ORIENTED_EDGE('',*,*,#3863,.F.);
#5245=ORIENTED_EDGE('',*,*,#3972,.T.);
#5246=ORIENTED_EDGE('',*,*,#3973,.T.);
#5247=ORIENTED_EDGE('',*,*,#3968,.F.);
#5248=ORIENTED_EDGE('',*,*,#3908,.T.);
#5249=ORIENTED_EDGE('',*,*,#3966,.F.);
#5250=ORIENTED_EDGE('',*,*,#3974,.T.);
#5251=ORIENTED_EDGE('',*,*,#3972,.F.);
#5252=ORIENTED_EDGE('',*,*,#3911,.T.);
#5253=ORIENTED_EDGE('',*,*,#3975,.T.);
#5254=ORIENTED_EDGE('',*,*,#3976,.T.);
#5255=ORIENTED_EDGE('',*,*,#3861,.F.);
#5256=ORIENTED_EDGE('',*,*,#3971,.T.);
#5257=ORIENTED_EDGE('',*,*,#3977,.T.);
#5258=ORIENTED_EDGE('',*,*,#3975,.F.);
#5259=ORIENTED_EDGE('',*,*,#3910,.T.);
#5260=ORIENTED_EDGE('',*,*,#3969,.F.);
#5261=ORIENTED_EDGE('',*,*,#3973,.F.);
#5262=ORIENTED_EDGE('',*,*,#3974,.F.);
#5263=ORIENTED_EDGE('',*,*,#3965,.F.);
#5264=ORIENTED_EDGE('',*,*,#3976,.F.);
#5265=ORIENTED_EDGE('',*,*,#3977,.F.);
#5266=ORIENTED_EDGE('',*,*,#3970,.F.);
#5267=ORIENTED_EDGE('',*,*,#3967,.F.);
#5268=ORIENTED_EDGE('',*,*,#3921,.F.);
#5269=ORIENTED_EDGE('',*,*,#3978,.T.);
#5270=ORIENTED_EDGE('',*,*,#3883,.T.);
#5271=ORIENTED_EDGE('',*,*,#3895,.T.);
#5272=ORIENTED_EDGE('',*,*,#3979,.T.);
#5273=ORIENTED_EDGE('',*,*,#3916,.F.);
#5274=ORIENTED_EDGE('',*,*,#3917,.F.);
#5275=ORIENTED_EDGE('',*,*,#3979,.F.);
#5276=ORIENTED_EDGE('',*,*,#3894,.F.);
#5277=ORIENTED_EDGE('',*,*,#3898,.F.);
#5278=ORIENTED_EDGE('',*,*,#3884,.F.);
#5279=ORIENTED_EDGE('',*,*,#3978,.F.);
#5280=ORIENTED_EDGE('',*,*,#3920,.F.);
#5281=ORIENTED_EDGE('',*,*,#3900,.F.);
#5282=ORIENTED_EDGE('',*,*,#3922,.F.);
#5283=ORIENTED_EDGE('',*,*,#3881,.F.);
#5284=ORIENTED_EDGE('',*,*,#3919,.F.);
#5285=ORIENTED_EDGE('',*,*,#3912,.F.);
#6450=TOROIDAL_SURFACE('',#7358,9.44563594905814,2.);
#6555=ADVANCED_FACE('',(#1903),#1685,.F.);
#6556=ADVANCED_FACE('',(#1904),#1686,.T.);
#6557=ADVANCED_FACE('',(#1905),#1687,.T.);
#6558=ADVANCED_FACE('',(#1906),#1688,.T.);
#6559=ADVANCED_FACE('',(#1907),#1689,.F.);
#6560=ADVANCED_FACE('',(#1908),#1690,.F.);
#6561=ADVANCED_FACE('',(#1909,#301,#302),#119,.T.);
#6562=ADVANCED_FACE('',(#1910),#1691,.F.);
#6563=ADVANCED_FACE('',(#1911),#441,.T.);
#6564=ADVANCED_FACE('',(#1912),#120,.T.);
#6565=ADVANCED_FACE('',(#1913,#303),#1692,.T.);
#6566=ADVANCED_FACE('',(#1914),#442,.T.);
#6567=ADVANCED_FACE('',(#1915,#304),#443,.T.);
#6568=ADVANCED_FACE('',(#1916,#305),#444,.T.);
#6569=ADVANCED_FACE('',(#1917),#445,.F.);
#6570=ADVANCED_FACE('',(#1918),#446,.F.);
#6571=ADVANCED_FACE('',(#1919,#306),#447,.F.);
#6572=ADVANCED_FACE('',(#1920),#448,.F.);
#6573=ADVANCED_FACE('',(#1921,#307),#449,.F.);
#6574=ADVANCED_FACE('',(#1922),#450,.F.);
#6575=ADVANCED_FACE('',(#1923),#451,.F.);
#6576=ADVANCED_FACE('',(#1924),#452,.T.);
#6577=ADVANCED_FACE('',(#1925),#453,.F.);
#6578=ADVANCED_FACE('',(#1926,#308),#454,.F.);
#6579=ADVANCED_FACE('',(#1927,#309),#455,.F.);
#6580=ADVANCED_FACE('',(#1928),#456,.T.);
#6581=ADVANCED_FACE('',(#1929),#457,.F.);
#6582=ADVANCED_FACE('',(#1930),#1693,.T.);
#6583=ADVANCED_FACE('',(#1931),#1694,.T.);
#6584=ADVANCED_FACE('',(#1932),#1695,.T.);
#6585=ADVANCED_FACE('',(#1933),#1696,.T.);
#6586=ADVANCED_FACE('',(#1934),#1697,.T.);
#6587=ADVANCED_FACE('',(#1935),#1698,.T.);
#6588=ADVANCED_FACE('',(#1936),#458,.F.);
#6589=ADVANCED_FACE('',(#1937,#310),#459,.T.);
#6590=ADVANCED_FACE('',(#1938),#460,.T.);
#6591=ADVANCED_FACE('',(#1939,#311),#461,.T.);
#6592=ADVANCED_FACE('',(#1940),#462,.T.);
#6593=ADVANCED_FACE('',(#1941),#1699,.T.);
#6594=ADVANCED_FACE('',(#1942),#1700,.T.);
#6595=ADVANCED_FACE('',(#1943),#1701,.F.);
#6596=ADVANCED_FACE('',(#1944),#1702,.F.);
#6597=ADVANCED_FACE('',(#1945),#1703,.T.);
#6598=ADVANCED_FACE('',(#1946),#1704,.T.);
#6599=ADVANCED_FACE('',(#1947),#6450,.T.);
#6845=CLOSED_SHELL('',(#6555,#6556,#6557,#6558,#6559,#6560,#6561,#6562,
#6563,#6564,#6565,#6566,#6567,#6568,#6569,#6570,#6571,#6572,#6573,#6574,
#6575,#6576,#6577,#6578,#6579,#6580,#6581,#6582,#6583,#6584,#6585,#6586,
#6587,#6588,#6589,#6590,#6591,#6592,#6593,#6594,#6595,#6596,#6597,#6598,
#6599));
#7274=AXIS2_PLACEMENT_3D('',#10586,#8381,#8382);
#7275=AXIS2_PLACEMENT_3D('',#10587,#8383,#8384);
#7276=AXIS2_PLACEMENT_3D('',#10589,#8385,#8386);
#7277=AXIS2_PLACEMENT_3D('',#10592,#8388,#8389);
#7278=AXIS2_PLACEMENT_3D('',#10593,#8390,#8391);
#7279=AXIS2_PLACEMENT_3D('',#10595,#8392,#8393);
#7280=AXIS2_PLACEMENT_3D('',#10598,#8395,#8396);
#7281=AXIS2_PLACEMENT_3D('',#10599,#8397,#8398);
#7282=AXIS2_PLACEMENT_3D('',#10601,#8399,#8400);
#7283=AXIS2_PLACEMENT_3D('',#10604,#8402,#8403);
#7284=AXIS2_PLACEMENT_3D('',#10605,#8404,#8405);
#7285=AXIS2_PLACEMENT_3D('',#10607,#8406,#8407);
#7286=AXIS2_PLACEMENT_3D('',#10610,#8409,#8410);
#7287=AXIS2_PLACEMENT_3D('',#10611,#8411,#8412);
#7288=AXIS2_PLACEMENT_3D('',#10613,#8413,#8414);
#7289=AXIS2_PLACEMENT_3D('',#10654,#8416,#8417);
#7290=AXIS2_PLACEMENT_3D('',#10677,#8419,#8420);
#7291=AXIS2_PLACEMENT_3D('',#10697,#8421,#8422);
#7292=AXIS2_PLACEMENT_3D('',#10700,#8423,#8424);
#7293=AXIS2_PLACEMENT_3D('',#10748,#8425,#8426);
#7294=AXIS2_PLACEMENT_3D('',#10797,#8428,#8429);
#7295=AXIS2_PLACEMENT_3D('',#10843,#8430,#8431);
#7296=AXIS2_PLACEMENT_3D('',#10846,#8432,#8433);
#7297=AXIS2_PLACEMENT_3D('',#10861,#8436,#8437);
#7298=AXIS2_PLACEMENT_3D('',#10863,#8439,#8440);
#7299=AXIS2_PLACEMENT_3D('',#10872,#8445,#8446);
#7300=AXIS2_PLACEMENT_3D('',#10873,#8447,#8448);
#7301=AXIS2_PLACEMENT_3D('',#10874,#8449,#8450);
#7302=AXIS2_PLACEMENT_3D('',#10879,#8452,#8453);
#7303=AXIS2_PLACEMENT_3D('',#10882,#8455,#8456);
#7304=AXIS2_PLACEMENT_3D('',#10883,#8457,#8458);
#7305=AXIS2_PLACEMENT_3D('',#10886,#8459,#8460);
#7306=AXIS2_PLACEMENT_3D('',#10892,#8464,#8465);
#7307=AXIS2_PLACEMENT_3D('',#10894,#8466,#8467);
#7308=AXIS2_PLACEMENT_3D('',#10895,#8468,#8469);
#7309=AXIS2_PLACEMENT_3D('',#10910,#8471,#8472);
#7310=AXIS2_PLACEMENT_3D('',#10912,#8473,#8474);
#7311=AXIS2_PLACEMENT_3D('',#10913,#8475,#8476);
#7312=AXIS2_PLACEMENT_3D('',#10928,#8478,#8479);
#7313=AXIS2_PLACEMENT_3D('',#10929,#8480,#8481);
#7314=AXIS2_PLACEMENT_3D('',#10935,#8485,#8486);
#7315=AXIS2_PLACEMENT_3D('',#10940,#8488,#8489);
#7316=AXIS2_PLACEMENT_3D('',#10946,#8493,#8494);
#7317=AXIS2_PLACEMENT_3D('',#10947,#8495,#8496);
#7318=AXIS2_PLACEMENT_3D('',#10951,#8499,#8500);
#7319=AXIS2_PLACEMENT_3D('',#10954,#8502,#8503);
#7320=AXIS2_PLACEMENT_3D('',#10956,#8504,#8505);
#7321=AXIS2_PLACEMENT_3D('',#10958,#8507,#8508);
#7322=AXIS2_PLACEMENT_3D('',#10968,#8514,#8515);
#7323=AXIS2_PLACEMENT_3D('',#10978,#8521,#8522);
#7324=AXIS2_PLACEMENT_3D('',#10984,#8526,#8527);
#7325=AXIS2_PLACEMENT_3D('',#10993,#8532,#8533);
#7326=AXIS2_PLACEMENT_3D('',#10994,#8534,#8535);
#7327=AXIS2_PLACEMENT_3D('',#10995,#8536,#8537);
#7328=AXIS2_PLACEMENT_3D('',#10996,#8538,#8539);
#7329=AXIS2_PLACEMENT_3D('',#10997,#8540,#8541);
#7330=AXIS2_PLACEMENT_3D('',#10998,#8542,#8543);
#7331=AXIS2_PLACEMENT_3D('',#10999,#8544,#8545);
#7332=AXIS2_PLACEMENT_3D('',#11000,#8546,#8547);
#7333=AXIS2_PLACEMENT_3D('',#11001,#8548,#8549);
#7334=AXIS2_PLACEMENT_3D('',#11002,#8550,#8551);
#7335=AXIS2_PLACEMENT_3D('',#11003,#8552,#8553);
#7336=AXIS2_PLACEMENT_3D('',#11004,#8554,#8555);
#7337=AXIS2_PLACEMENT_3D('',#11005,#8556,#8557);
#7338=AXIS2_PLACEMENT_3D('',#11006,#8558,#8559);
#7339=AXIS2_PLACEMENT_3D('',#11007,#8560,#8561);
#7340=AXIS2_PLACEMENT_3D('',#11008,#8562,#8563);
#7341=AXIS2_PLACEMENT_3D('',#11009,#8564,#8565);
#7342=AXIS2_PLACEMENT_3D('',#11010,#8566,#8567);
#7343=AXIS2_PLACEMENT_3D('',#11011,#8568,#8569);
#7344=AXIS2_PLACEMENT_3D('',#11020,#8574,#8575);
#7345=AXIS2_PLACEMENT_3D('',#11023,#8577,#8578);
#7346=AXIS2_PLACEMENT_3D('',#11025,#8579,#8580);
#7347=AXIS2_PLACEMENT_3D('',#11027,#8582,#8583);
#7348=AXIS2_PLACEMENT_3D('',#11031,#8586,#8587);
#7349=AXIS2_PLACEMENT_3D('',#11032,#8588,#8589);
#7350=AXIS2_PLACEMENT_3D('',#11035,#8591,#8592);
#7351=AXIS2_PLACEMENT_3D('',#11036,#8593,#8594);
#7352=AXIS2_PLACEMENT_3D('',#11038,#8596,#8597);
#7353=AXIS2_PLACEMENT_3D('',#11039,#8598,#8599);
#7354=AXIS2_PLACEMENT_3D('',#11040,#8600,#8601);
#7355=AXIS2_PLACEMENT_3D('',#11042,#8603,#8604);
#7356=AXIS2_PLACEMENT_3D('',#11044,#8606,#8607);
#7357=AXIS2_PLACEMENT_3D('',#11045,#8608,#8609);
#7358=AXIS2_PLACEMENT_3D('',#11046,#8610,#8611);
#8381=DIRECTION('axis',(0.,0.,1.));
#8382=DIRECTION('refdir',(1.,0.,0.));
#8383=DIRECTION('center_axis',(0.,-1.,0.));
#8384=DIRECTION('ref_axis',(0.,0.,-1.));
#8385=DIRECTION('center_axis',(0.,1.,0.));
#8386=DIRECTION('ref_axis',(0.,0.,1.));
#8387=DIRECTION('',(0.,-1.,0.));
#8388=DIRECTION('center_axis',(0.,-1.,0.));
#8389=DIRECTION('ref_axis',(0.,0.,-1.));
#8390=DIRECTION('center_axis',(0.,1.,0.));
#8391=DIRECTION('ref_axis',(0.,0.,1.));
#8392=DIRECTION('center_axis',(0.,-1.,0.));
#8393=DIRECTION('ref_axis',(0.,0.,-1.));
#8394=DIRECTION('',(0.,-1.,0.));
#8395=DIRECTION('center_axis',(0.,1.,0.));
#8396=DIRECTION('ref_axis',(0.,0.,-1.));
#8397=DIRECTION('center_axis',(0.,1.,0.));
#8398=DIRECTION('ref_axis',(0.,0.,1.));
#8399=DIRECTION('center_axis',(0.,-1.,0.));
#8400=DIRECTION('ref_axis',(0.,0.,1.));
#8401=DIRECTION('',(0.,-1.,0.));
#8402=DIRECTION('center_axis',(0.,-1.,0.));
#8403=DIRECTION('ref_axis',(0.,0.,-1.));
#8404=DIRECTION('center_axis',(0.,1.,0.));
#8405=DIRECTION('ref_axis',(0.,0.,1.));
#8406=DIRECTION('center_axis',(0.,-1.,0.));
#8407=DIRECTION('ref_axis',(0.,0.,1.));
#8408=DIRECTION('',(0.,-1.,0.));
#8409=DIRECTION('center_axis',(0.,1.,0.));
#8410=DIRECTION('ref_axis',(0.,0.,-1.));
#8411=DIRECTION('center_axis',(0.,-1.,0.));
#8412=DIRECTION('ref_axis',(0.,0.,-1.));
#8413=DIRECTION('center_axis',(0.,-1.,-1.24352412568707E-16));
#8414=DIRECTION('ref_axis',(0.,-1.24352412568707E-16,1.));
#8415=DIRECTION('',(0.,-1.,0.));
#8416=DIRECTION('center_axis',(0.,-1.,0.));
#8417=DIRECTION('ref_axis',(0.,0.,-1.));
#8418=DIRECTION('',(0.,-1.,0.));
#8419=DIRECTION('center_axis',(0.,1.,1.24352412568707E-16));
#8420=DIRECTION('ref_axis',(0.,1.24352412568707E-16,-1.));
#8421=DIRECTION('center_axis',(0.,0.,-1.));
#8422=DIRECTION('ref_axis',(1.,0.,0.));
#8423=DIRECTION('center_axis',(0.,0.,1.));
#8424=DIRECTION('ref_axis',(-1.,1.77635684682688E-15,0.));
#8425=DIRECTION('center_axis',(0.,0.,1.));
#8426=DIRECTION('ref_axis',(-1.,0.,0.));
#8427=DIRECTION('',(0.0174524064372835,-2.1373033680838E-18,0.999847695156391));
#8428=DIRECTION('center_axis',(0.,0.,1.));
#8429=DIRECTION('ref_axis',(-1.,0.,0.));
#8430=DIRECTION('center_axis',(0.,-1.,0.));
#8431=DIRECTION('ref_axis',(0.,0.,-1.));
#8432=DIRECTION('center_axis',(0.,1.,1.24352412568707E-16));
#8433=DIRECTION('ref_axis',(0.,-1.24352412568707E-16,1.));
#8434=DIRECTION('',(0.,-1.,0.));
#8435=DIRECTION('',(0.,-1.,0.));
#8436=DIRECTION('center_axis',(0.,-1.,-1.24352412568707E-16));
#8437=DIRECTION('ref_axis',(0.,1.24352412568707E-16,-1.));
#8438=DIRECTION('',(0.,1.,0.));
#8439=DIRECTION('center_axis',(-0.707106781186547,0.,-0.707106781186548));
#8440=DIRECTION('ref_axis',(-0.707106781186548,0.,0.707106781186547));
#8441=DIRECTION('',(-0.707106781186548,0.,0.707106781186547));
#8442=DIRECTION('',(0.,1.,0.));
#8443=DIRECTION('',(-0.707106781186548,0.,0.707106781186547));
#8444=DIRECTION('',(0.,-1.,0.));
#8445=DIRECTION('center_axis',(0.,0.,-1.));
#8446=DIRECTION('ref_axis',(-1.,-1.22464679914735E-16,0.));
#8447=DIRECTION('center_axis',(0.,0.,-1.));
#8448=DIRECTION('ref_axis',(1.,1.77635684759209E-15,0.));
#8449=DIRECTION('center_axis',(0.,-1.,0.));
#8450=DIRECTION('ref_axis',(3.0760962761356E-5,0.,0.999999999526882));
#8451=DIRECTION('',(0.,1.,0.));
#8452=DIRECTION('center_axis',(0.,1.,0.));
#8453=DIRECTION('ref_axis',(0.,0.,-1.));
#8454=DIRECTION('',(0.,-1.,0.));
#8455=DIRECTION('center_axis',(0.,-1.,0.));
#8456=DIRECTION('ref_axis',(0.,0.,1.));
#8457=DIRECTION('center_axis',(0.,1.15648231731787E-16,-1.));
#8458=DIRECTION('ref_axis',(0.,1.,1.15648231731787E-16));
#8459=DIRECTION('center_axis',(0.,1.15648231731787E-16,-1.));
#8460=DIRECTION('ref_axis',(0.,1.,1.15648231731787E-16));
#8461=DIRECTION('',(-1.,0.,0.));
#8462=DIRECTION('',(0.,-1.,-1.15648231731787E-16));
#8463=DIRECTION('',(-1.,0.,0.));
#8464=DIRECTION('center_axis',(0.,1.,1.24352412568707E-16));
#8465=DIRECTION('ref_axis',(0.,-1.24352412568707E-16,1.));
#8466=DIRECTION('center_axis',(0.,-1.,-1.24352412568707E-16));
#8467=DIRECTION('ref_axis',(0.,-1.24352412568707E-16,1.));
#8468=DIRECTION('center_axis',(0.,1.,1.24352412568707E-16));
#8469=DIRECTION('ref_axis',(0.,-1.24352412568707E-16,1.));
#8470=DIRECTION('',(0.,1.24352412568707E-16,-1.));
#8471=DIRECTION('center_axis',(0.,-1.,-1.24352412568707E-16));
#8472=DIRECTION('ref_axis',(0.,1.24352412568707E-16,-1.));
#8473=DIRECTION('center_axis',(0.,-1.,-1.24352412568707E-16));
#8474=DIRECTION('ref_axis',(0.,1.24352412568707E-16,-1.));
#8475=DIRECTION('center_axis',(0.,1.,1.24352412568707E-16));
#8476=DIRECTION('ref_axis',(0.,1.24352412568707E-16,-1.));
#8477=DIRECTION('',(0.,-1.24352412568707E-16,1.));
#8478=DIRECTION('center_axis',(-1.,0.,0.));
#8479=DIRECTION('ref_axis',(0.,0.,1.));
#8480=DIRECTION('center_axis',(0.,0.,1.));
#8481=DIRECTION('ref_axis',(1.,0.,0.));
#8482=DIRECTION('',(-1.,0.,0.));
#8483=DIRECTION('',(0.,1.,0.));
#8484=DIRECTION('',(-1.,0.,0.));
#8485=DIRECTION('center_axis',(0.,-1.,0.));
#8486=DIRECTION('ref_axis',(0.,0.,-1.));
#8487=DIRECTION('',(0.707106781186548,0.,-0.707106781186547));
#8488=DIRECTION('center_axis',(0.,1.,0.));
#8489=DIRECTION('ref_axis',(0.,0.,-1.));
#8490=DIRECTION('',(0.707106781186548,0.,0.707106781186548));
#8491=DIRECTION('',(-1.,0.,0.));
#8492=DIRECTION('',(0.707106781186548,0.,0.707106781186548));
#8493=DIRECTION('center_axis',(0.,1.,0.));
#8494=DIRECTION('ref_axis',(-7.70988211545247E-15,0.,-1.));
#8495=DIRECTION('center_axis',(0.,0.,-1.));
#8496=DIRECTION('ref_axis',(-1.,0.,0.));
#8497=DIRECTION('',(0.,-1.,0.));
#8498=DIRECTION('',(-1.,0.,0.));
#8499=DIRECTION('center_axis',(0.,1.,0.));
#8500=DIRECTION('ref_axis',(0.,0.,1.));
#8501=DIRECTION('',(0.707106781186548,0.,0.707106781186548));
#8502=DIRECTION('center_axis',(0.,-1.,0.));
#8503=DIRECTION('ref_axis',(-3.85494105772624E-15,0.,1.));
#8504=DIRECTION('center_axis',(0.,-1.,0.));
#8505=DIRECTION('ref_axis',(3.85494105772624E-15,0.,1.));
#8506=DIRECTION('',(0.707106781186548,0.,0.707106781186548));
#8507=DIRECTION('center_axis',(-0.707106781186548,0.,0.707106781186547));
#8508=DIRECTION('ref_axis',(0.707106781186547,0.,0.707106781186548));
#8509=DIRECTION('',(0.,1.,0.));
#8510=DIRECTION('',(0.707106781186547,0.,0.707106781186548));
#8511=DIRECTION('',(0.,1.,0.));
#8512=DIRECTION('',(-0.707106781186547,0.,-0.707106781186548));
#8513=DIRECTION('',(0.,1.,0.));
#8514=DIRECTION('center_axis',(0.707106781186548,0.,-0.707106781186547));
#8515=DIRECTION('ref_axis',(-0.707106781186547,0.,-0.707106781186548));
#8516=DIRECTION('',(-0.707106781186547,0.,-0.707106781186548));
#8517=DIRECTION('',(0.,-1.,0.));
#8518=DIRECTION('',(0.707106781186547,0.,0.707106781186548));
#8519=DIRECTION('',(0.,-1.,0.));
#8520=DIRECTION('',(0.,-1.,0.));
#8521=DIRECTION('center_axis',(-0.707106781186547,0.,-0.707106781186548));
#8522=DIRECTION('ref_axis',(-0.707106781186548,0.,0.707106781186547));
#8523=DIRECTION('',(0.707106781186548,0.,-0.707106781186547));
#8524=DIRECTION('',(0.,1.,0.));
#8525=DIRECTION('',(0.,-1.,0.));
#8526=DIRECTION('center_axis',(0.707106781186548,0.,0.707106781186548));
#8527=DIRECTION('ref_axis',(0.707106781186548,0.,-0.707106781186548));
#8528=DIRECTION('',(-0.707106781186547,0.,0.707106781186547));
#8529=DIRECTION('',(0.,1.,0.));
#8530=DIRECTION('',(-0.707106781186547,0.,0.707106781186547));
#8531=DIRECTION('',(0.,-1.,0.));
#8532=DIRECTION('center_axis',(0.,-1.,0.));
#8533=DIRECTION('ref_axis',(0.,0.,-1.));
#8534=DIRECTION('center_axis',(0.,1.,0.));
#8535=DIRECTION('ref_axis',(0.,0.,-1.));
#8536=DIRECTION('center_axis',(0.,-1.,0.));
#8537=DIRECTION('ref_axis',(0.,0.,-1.));
#8538=DIRECTION('center_axis',(0.,-1.,0.));
#8539=DIRECTION('ref_axis',(0.,0.,-1.));
#8540=DIRECTION('center_axis',(0.,1.,0.));
#8541=DIRECTION('ref_axis',(-7.70988211545247E-15,0.,-1.));
#8542=DIRECTION('center_axis',(0.,1.,0.));
#8543=DIRECTION('ref_axis',(0.,0.,1.));
#8544=DIRECTION('center_axis',(0.,-1.,0.));
#8545=DIRECTION('ref_axis',(3.85494105772624E-15,0.,1.));
#8546=DIRECTION('center_axis',(0.,-1.,0.));
#8547=DIRECTION('ref_axis',(3.85494105772624E-15,0.,1.));
#8548=DIRECTION('center_axis',(0.,1.,0.));
#8549=DIRECTION('ref_axis',(0.,0.,1.));
#8550=DIRECTION('center_axis',(0.,1.,0.));
#8551=DIRECTION('ref_axis',(0.,0.,1.));
#8552=DIRECTION('center_axis',(0.,-1.,0.));
#8553=DIRECTION('ref_axis',(0.,0.,-1.));
#8554=DIRECTION('center_axis',(0.,-1.,0.));
#8555=DIRECTION('ref_axis',(0.,0.,-1.));
#8556=DIRECTION('center_axis',(0.,1.,0.));
#8557=DIRECTION('ref_axis',(0.,0.,1.));
#8558=DIRECTION('center_axis',(0.,-1.,0.));
#8559=DIRECTION('ref_axis',(0.,0.,-1.));
#8560=DIRECTION('center_axis',(0.,-1.,0.));
#8561=DIRECTION('ref_axis',(0.,0.,-1.));
#8562=DIRECTION('center_axis',(0.,1.,0.));
#8563=DIRECTION('ref_axis',(1.22464679914735E-16,0.,-1.));
#8564=DIRECTION('center_axis',(0.,1.,0.));
#8565=DIRECTION('ref_axis',(1.22464679914735E-16,0.,-1.));
#8566=DIRECTION('center_axis',(0.,1.,0.));
#8567=DIRECTION('ref_axis',(1.01064309961486E-15,0.,-1.));
#8568=DIRECTION('center_axis',(0.,0.,-1.));
#8569=DIRECTION('ref_axis',(-1.,0.,0.));
#8570=DIRECTION('',(1.,0.,0.));
#8571=DIRECTION('',(0.,1.,0.));
#8572=DIRECTION('',(-1.,0.,0.));
#8573=DIRECTION('',(0.,-1.,0.));
#8574=DIRECTION('center_axis',(0.,-1.,0.));
#8575=DIRECTION('ref_axis',(0.,0.,-1.));
#8576=DIRECTION('',(0.,0.,1.));
#8577=DIRECTION('center_axis',(0.,-1.,0.));
#8578=DIRECTION('ref_axis',(0.,0.,-1.));
#8579=DIRECTION('center_axis',(0.,-1.,0.));
#8580=DIRECTION('ref_axis',(0.,0.,-1.));
#8581=DIRECTION('',(0.,0.,1.));
#8582=DIRECTION('center_axis',(1.,0.,0.));
#8583=DIRECTION('ref_axis',(0.,0.,-1.));
#8584=DIRECTION('',(0.,0.,1.));
#8585=DIRECTION('',(0.,-1.,0.));
#8586=DIRECTION('center_axis',(0.,1.,0.));
#8587=DIRECTION('ref_axis',(0.,0.,1.));
#8588=DIRECTION('center_axis',(0.,1.,0.));
#8589=DIRECTION('ref_axis',(0.,0.,1.));
#8590=DIRECTION('',(0.,0.,1.));
#8591=DIRECTION('center_axis',(0.,1.,0.));
#8592=DIRECTION('ref_axis',(0.,0.,1.));
#8593=DIRECTION('center_axis',(-1.,0.,0.));
#8594=DIRECTION('ref_axis',(0.,0.,1.));
#8595=DIRECTION('',(0.,1.,0.));
#8596=DIRECTION('center_axis',(0.,-1.,0.));
#8597=DIRECTION('ref_axis',(0.,0.,-1.));
#8598=DIRECTION('center_axis',(0.,1.,0.));
#8599=DIRECTION('ref_axis',(0.,0.,1.));
#8600=DIRECTION('center_axis',(0.,-1.,0.));
#8601=DIRECTION('ref_axis',(0.,0.,-1.));
#8602=DIRECTION('',(0.,1.,0.));
#8603=DIRECTION('center_axis',(0.,-1.,0.));
#8604=DIRECTION('ref_axis',(0.,0.,-1.));
#8605=DIRECTION('',(0.,1.,0.));
#8606=DIRECTION('center_axis',(0.,-1.,0.));
#8607=DIRECTION('ref_axis',(0.,0.,-1.));
#8608=DIRECTION('center_axis',(0.,-1.,0.));
#8609=DIRECTION('ref_axis',(0.,0.,-1.));
#8610=DIRECTION('center_axis',(0.,1.15648231731787E-16,-1.));
#8611=DIRECTION('ref_axis',(0.,1.,0.));
#10586=CARTESIAN_POINT('',(0.,0.,0.));
#10587=CARTESIAN_POINT('Origin',(-0.414990954321311,5.02189031698537,38.8542865365866));
#10588=CARTESIAN_POINT('',(-0.414990954321311,3.97811209444304,40.2042865365866));
#10589=CARTESIAN_POINT('Origin',(-0.414990954321311,3.97811209444304,38.8542865365866));
#10590=CARTESIAN_POINT('',(-0.414990954321311,-3.97810968301463,40.2042865365866));
#10591=CARTESIAN_POINT('',(-0.414990954321311,5.02189031698537,40.2042865365866));
#10592=CARTESIAN_POINT('Origin',(-0.414990954321311,-3.97810968301463,38.8542865365866));
#10593=CARTESIAN_POINT('Origin',(-16.3206772921779,-4.87810968301463,0.853093602568413));
#10594=CARTESIAN_POINT('',(-16.3206772921779,4.87789031698537,-0.0469063974315885));
#10595=CARTESIAN_POINT('Origin',(-16.3206772921779,4.87789031698537,0.853093602568413));
#10596=CARTESIAN_POINT('',(-16.3206772921779,3.97811209444304,-0.0469063974315885));
#10597=CARTESIAN_POINT('',(-16.3206772921779,-4.87810968301463,-0.0469063974315885));
#10598=CARTESIAN_POINT('Origin',(-16.3206772921779,3.97811209444304,0.853093602568413));
#10599=CARTESIAN_POINT('Origin',(-16.3206772921779,-4.87810968301463,0.853093602568413));
#10600=CARTESIAN_POINT('',(-16.3206772921779,-3.97810968301463,-0.0469063974315885));
#10601=CARTESIAN_POINT('Origin',(-16.3206772921779,-3.97810968301463,0.853093602568413));
#10602=CARTESIAN_POINT('',(-16.3206772921779,-4.87810968301463,-0.0469063974315885));
#10603=CARTESIAN_POINT('',(-16.3206772921779,-4.87810968301463,-0.0469063974315885));
#10604=CARTESIAN_POINT('Origin',(-16.3206772921779,-4.87810968301463,0.853093602568413));
#10605=CARTESIAN_POINT('Origin',(-16.3206772921779,-4.87810968301463,0.853093602568413));
#10606=CARTESIAN_POINT('',(-16.3206772921779,2.2500012057142,-0.0469063974315885));
#10607=CARTESIAN_POINT('Origin',(-16.3206772921779,2.2500012057142,0.853093602568413));
#10608=CARTESIAN_POINT('',(-16.3206772921779,-2.2499987942858,-0.0469063974315885));
#10609=CARTESIAN_POINT('',(-16.3206772921779,-4.87810968301463,-0.0469063974315885));
#10610=CARTESIAN_POINT('Origin',(-16.3206772921779,-2.2499987942858,0.853093602568413));
#10611=CARTESIAN_POINT('Origin',(-0.0886968229780924,16.2000012057142,10.3078072726059));
#10612=CARTESIAN_POINT('',(-0.0886968229780925,-6.74999879428579,11.6578072726059));
#10613=CARTESIAN_POINT('Origin',(-0.0886968229780924,-6.7499987942858,10.3078072726059));
#10614=CARTESIAN_POINT('',(-0.0886968229780923,-11.5362972391425,11.6578072726059));
#10615=CARTESIAN_POINT('',(-0.0886968229780925,16.2000012057142,11.6578072726059));
#10616=CARTESIAN_POINT('',(-0.0886968229780924,-11.5834259144487,8.95780727260587));
#10617=CARTESIAN_POINT('Ctrl Pts',(-0.0886968229780924,-11.5362972391425,
11.6578072726059));
#10618=CARTESIAN_POINT('Ctrl Pts',(-0.25812669739265,-11.5362972391425,
11.6578072726059));
#10619=CARTESIAN_POINT('Ctrl Pts',(-0.438786097024996,-11.5327733929255,
11.6239637415438));
#10620=CARTESIAN_POINT('Ctrl Pts',(-0.771068298404367,-11.5202944277784,
11.4864503548939));
#10621=CARTESIAN_POINT('Ctrl Pts',(-0.922701599335139,-11.5115497231097,
11.3827868553843));
#10622=CARTESIAN_POINT('Ctrl Pts',(-1.16219358624327,-11.4958808036504,
11.1437012818572));
#10623=CARTESIAN_POINT('Ctrl Pts',(-1.26609750553296,-11.4879422226462,
10.9923037050953));
#10624=CARTESIAN_POINT('Ctrl Pts',(-1.40417808237572,-11.4787820664037,
10.6603931046871));
#10625=CARTESIAN_POINT('Ctrl Pts',(-1.43834888045985,-11.4777789903649,
10.4798716492407));
#10626=CARTESIAN_POINT('Ctrl Pts',(-1.43904053671719,-11.4836610089555,
10.1405693130855));
#10627=CARTESIAN_POINT('Ctrl Pts',(-1.40534901915338,-11.4909660193735,
9.95937865043048));
#10628=CARTESIAN_POINT('Ctrl Pts',(-1.26785312558251,-11.5117339111722,
9.6262165078671));
#10629=CARTESIAN_POINT('Ctrl Pts',(-1.16405939063838,-11.5249769926622,
9.47422697160051));
#10630=CARTESIAN_POINT('Ctrl Pts',(-0.924500341537122,-11.549023167757,
9.23417909181128));
#10631=CARTESIAN_POINT('Ctrl Pts',(-0.772719647754745,-11.5614014702908,
9.13005765427303));
#10632=CARTESIAN_POINT('Ctrl Pts',(-0.439810200113418,-11.5787081985477,
8.99186624382722));
#10633=CARTESIAN_POINT('Ctrl Pts',(-0.258665959021164,-11.5834259144487,
8.95780727260587));
#10634=CARTESIAN_POINT('Ctrl Pts',(-0.0886968229780923,-11.5834259144487,
8.95780727260587));
#10635=CARTESIAN_POINT('Ctrl Pts',(-0.0886968229780924,-11.5834259144487,
8.95780727260587));
#10636=CARTESIAN_POINT('Ctrl Pts',(0.0812723130649798,-11.5834259144487,
8.95780727260587));
#10637=CARTESIAN_POINT('Ctrl Pts',(0.262416554157233,-11.5787081985477,
8.99186624382722));
#10638=CARTESIAN_POINT('Ctrl Pts',(0.595326001798561,-11.5614014702908,
9.13005765427303));
#10639=CARTESIAN_POINT('Ctrl Pts',(0.747106695580938,-11.549023167757,9.23417909181128));
#10640=CARTESIAN_POINT('Ctrl Pts',(0.986665744682193,-11.5249769926622,
9.47422697160051));
#10641=CARTESIAN_POINT('Ctrl Pts',(1.09045947962633,-11.5117339111722,9.6262165078671));
#10642=CARTESIAN_POINT('Ctrl Pts',(1.22795537319719,-11.4909660193735,9.95937865043048));
#10643=CARTESIAN_POINT('Ctrl Pts',(1.261646890761,-11.4836610089555,10.1405693130855));
#10644=CARTESIAN_POINT('Ctrl Pts',(1.26130037217385,-11.4807141278278,10.3105591959141));
#10645=CARTESIAN_POINT('Ctrl Pts',(1.26095523450366,-11.4777789903649,10.4798716492407));
#10646=CARTESIAN_POINT('Ctrl Pts',(1.22678443641954,-11.4787820664037,10.6603931046871));
#10647=CARTESIAN_POINT('Ctrl Pts',(1.08870385957678,-11.4879422226462,10.9923037050953));
#10648=CARTESIAN_POINT('Ctrl Pts',(0.984799940287087,-11.4958808036504,
11.1437012818572));
#10649=CARTESIAN_POINT('Ctrl Pts',(0.745307953378954,-11.5115497231097,
11.3827868553843));
#10650=CARTESIAN_POINT('Ctrl Pts',(0.593674652448182,-11.5202944277784,
11.4864503548939));
#10651=CARTESIAN_POINT('Ctrl Pts',(0.26139245106881,-11.5327733929255,11.6239637415438));
#10652=CARTESIAN_POINT('Ctrl Pts',(0.0807330514364638,-11.5362972391425,
11.6578072726059));
#10653=CARTESIAN_POINT('Ctrl Pts',(-0.0886968229780931,-11.5362972391425,
11.6578072726059));
#10654=CARTESIAN_POINT('Origin',(-0.0886968229780924,16.2000012057142,10.3078072726059));
#10655=CARTESIAN_POINT('',(-0.088696822977779,11.5834283258775,8.95780727260271));
#10656=CARTESIAN_POINT('',(-0.0886968229780923,11.5362996505709,11.6578072726059));
#10657=CARTESIAN_POINT('Ctrl Pts',(-0.0886968229780926,11.5834283258771,
8.95780727260587));
#10658=CARTESIAN_POINT('Ctrl Pts',(-0.258665959021165,11.5834283258771,
8.95780727260587));
#10659=CARTESIAN_POINT('Ctrl Pts',(-0.439810200113418,11.5787106099761,
8.99186624382722));
#10660=CARTESIAN_POINT('Ctrl Pts',(-0.772719647754746,11.5614038817192,
9.13005765427303));
#10661=CARTESIAN_POINT('Ctrl Pts',(-0.924500341537123,11.5490255791854,
9.23417909181128));
#10662=CARTESIAN_POINT('Ctrl Pts',(-1.16405939063838,11.5249794040906,9.47422697160051));
#10663=CARTESIAN_POINT('Ctrl Pts',(-1.26785312558251,11.5117363226006,9.6262165078671));
#10664=CARTESIAN_POINT('Ctrl Pts',(-1.40534901915338,11.4909684308019,9.95937865043048));
#10665=CARTESIAN_POINT('Ctrl Pts',(-1.43904053671719,11.4836634203839,10.1405693130855));
#10666=CARTESIAN_POINT('Ctrl Pts',(-1.43834888045985,11.4777814017933,10.4798716492407));
#10667=CARTESIAN_POINT('Ctrl Pts',(-1.40417808237572,11.4787844778321,10.6603931046871));
#10668=CARTESIAN_POINT('Ctrl Pts',(-1.26609750553296,11.4879446340746,10.9923037050953));
#10669=CARTESIAN_POINT('Ctrl Pts',(-1.16219358624327,11.4958832150788,11.1437012818572));
#10670=CARTESIAN_POINT('Ctrl Pts',(-0.922701599335138,11.5115521345381,
11.3827868553843));
#10671=CARTESIAN_POINT('Ctrl Pts',(-0.771068298404366,11.5202968392069,
11.4864503548939));
#10672=CARTESIAN_POINT('Ctrl Pts',(-0.438786097024993,11.5327758043539,
11.6239637415438));
#10673=CARTESIAN_POINT('Ctrl Pts',(-0.258126697392649,11.5362996505709,
11.6578072726059));
#10674=CARTESIAN_POINT('Ctrl Pts',(-0.088696822978092,11.5362996505709,
11.6578072726059));
#10675=CARTESIAN_POINT('',(-0.0886968229780925,6.7500012057142,11.6578072726059));
#10676=CARTESIAN_POINT('',(-0.0886968229780925,16.2000012057142,11.6578072726059));
#10677=CARTESIAN_POINT('Origin',(-0.0886968229780924,6.7500012057142,10.3078072726059));
#10678=CARTESIAN_POINT('Ctrl Pts',(-0.0886968229780922,11.5362996505709,
11.6578072726059));
#10679=CARTESIAN_POINT('Ctrl Pts',(0.0807330514364649,11.5362996505709,
11.6578072726059));
#10680=CARTESIAN_POINT('Ctrl Pts',(0.26139245106881,11.5327758043539,11.6239637415438));
#10681=CARTESIAN_POINT('Ctrl Pts',(0.593674652448182,11.5202968392069,11.4864503548939));
#10682=CARTESIAN_POINT('Ctrl Pts',(0.745307953378954,11.5115521345381,11.3827868553843));
#10683=CARTESIAN_POINT('Ctrl Pts',(0.984799940287087,11.4958832150788,11.1437012818572));
#10684=CARTESIAN_POINT('Ctrl Pts',(1.08870385957678,11.4879446340746,10.9923037050953));
#10685=CARTESIAN_POINT('Ctrl Pts',(1.22678443641954,11.4787844778321,10.6603931046871));
#10686=CARTESIAN_POINT('Ctrl Pts',(1.26095523450366,11.4777814017933,10.4798716492407));
#10687=CARTESIAN_POINT('Ctrl Pts',(1.26130037217385,11.4807165392562,10.3105591959141));
#10688=CARTESIAN_POINT('Ctrl Pts',(1.261646890761,11.4836634203839,10.1405693130855));
#10689=CARTESIAN_POINT('Ctrl Pts',(1.22795537319719,11.4909684308019,9.95937865043048));
#10690=CARTESIAN_POINT('Ctrl Pts',(1.09045947962633,11.5117363226006,9.6262165078671));
#10691=CARTESIAN_POINT('Ctrl Pts',(0.986665744682193,11.5249794040906,9.47422697160051));
#10692=CARTESIAN_POINT('Ctrl Pts',(0.747106695580938,11.5490255791854,9.23417909181128));
#10693=CARTESIAN_POINT('Ctrl Pts',(0.595326001798561,11.5614038817192,9.13005765427303));
#10694=CARTESIAN_POINT('Ctrl Pts',(0.262416554157233,11.5787106099761,8.99186624382722));
#10695=CARTESIAN_POINT('Ctrl Pts',(0.0812723130649793,11.5834283258771,
8.95780727260587));
#10696=CARTESIAN_POINT('Ctrl Pts',(-0.0886968229780928,11.5834283258771,
8.95780727260587));
#10697=CARTESIAN_POINT('Origin',(-0.0886968229780924,1.20571420388653E-6,
2.2793514595497));
#10698=CARTESIAN_POINT('',(9.15430644803649,-6.7499987942858,16.869309255546));
#10699=CARTESIAN_POINT('',(9.15430644803649,6.7500012057142,16.8693092555461));
#10700=CARTESIAN_POINT('Origin',(-0.0886968229780924,1.20571420052696E-6,
16.869309255546));
#10701=CARTESIAN_POINT('',(9.21661950459473,6.7500012057142,13.9829593621724));
#10702=CARTESIAN_POINT('Ctrl Pts',(9.21661950459473,6.7500012057142,13.9829593621724));
#10703=CARTESIAN_POINT('Ctrl Pts',(9.19587255806943,6.7500012057142,14.9450765126902));
#10704=CARTESIAN_POINT('Ctrl Pts',(9.17510170146439,6.7500012057142,15.9071931479242));
#10705=CARTESIAN_POINT('Ctrl Pts',(9.15430644803649,6.7500012057142,16.8693092555461));
#10706=CARTESIAN_POINT('',(3.79009320173104,10.9021010231549,9.63818989051917));
#10707=CARTESIAN_POINT('Ctrl Pts',(3.79009320173104,10.9021010231549,9.63818989051917));
#10708=CARTESIAN_POINT('Ctrl Pts',(4.20613537995868,10.7443331834893,10.1642783227575));
#10709=CARTESIAN_POINT('Ctrl Pts',(4.64694412836354,10.5510444035147,10.650798216911));
#10710=CARTESIAN_POINT('Ctrl Pts',(5.63962932833512,10.0329253784985,11.623427806388));
#10711=CARTESIAN_POINT('Ctrl Pts',(6.25376498977623,9.65635758742349,12.1401590568172));
#10712=CARTESIAN_POINT('Ctrl Pts',(7.45983969473753,8.72586417187042,13.0128149073975));
#10713=CARTESIAN_POINT('Ctrl Pts',(8.04927182637234,8.17020873374597,13.3703563763539));
#10714=CARTESIAN_POINT('Ctrl Pts',(8.77823970806682,7.33062511965669,13.765805640045));
#10715=CARTESIAN_POINT('Ctrl Pts',(9.0022731985786,7.04855860769825,13.8797875988384));
#10716=CARTESIAN_POINT('Ctrl Pts',(9.21661950459473,6.7500012057142,13.9829593621724));
#10717=CARTESIAN_POINT('',(-2.04522493875568,11.4685794314074,6.04489666046755));
#10718=CARTESIAN_POINT('Ctrl Pts',(3.79009320173104,10.9021010231549,9.63818989051918));
#10719=CARTESIAN_POINT('Ctrl Pts',(3.58403350493312,10.9802411611199,9.37762586958811));
#10720=CARTESIAN_POINT('Ctrl Pts',(3.36708944887808,11.0552744978014,9.13007814566772));
#10721=CARTESIAN_POINT('Ctrl Pts',(2.72899476230882,11.2526099540629,8.46885648760705));
#10722=CARTESIAN_POINT('Ctrl Pts',(2.23455214075372,11.3774728044186,8.03794303289295));
#10723=CARTESIAN_POINT('Ctrl Pts',(1.16082935689865,11.55806672261,7.28307730157583));
#10724=CARTESIAN_POINT('Ctrl Pts',(0.581234136539683,11.6122856652571,6.9592121964347));
#10725=CARTESIAN_POINT('Ctrl Pts',(-0.617178694535791,11.6334215213611,
6.42377887019057));
#10726=CARTESIAN_POINT('Ctrl Pts',(-1.32470976378382,11.5888829746167,6.19261208415742));
#10727=CARTESIAN_POINT('Ctrl Pts',(-2.04522493875569,11.4685794314074,6.04489666046755));
#10728=CARTESIAN_POINT('',(-11.0841037493982,3.97811118728989,2.68507615460814));
#10729=CARTESIAN_POINT('Ctrl Pts',(-11.0841037493982,3.97811118728989,2.68507615460814));
#10730=CARTESIAN_POINT('Ctrl Pts',(-11.0229709537136,4.14532830143922,2.71923525419231));
#10731=CARTESIAN_POINT('Ctrl Pts',(-10.9580372989578,4.31099505858238,2.75525104909031));
#10732=CARTESIAN_POINT('Ctrl Pts',(-10.2946364808206,5.8956035577366,3.11981222038323));
#10733=CARTESIAN_POINT('Ctrl Pts',(-9.4105044355921,7.17556183564993,3.57669501792371));
#10734=CARTESIAN_POINT('Ctrl Pts',(-7.37826383459281,9.21886256467337,4.47105415851211));
#10735=CARTESIAN_POINT('Ctrl Pts',(-6.07582291747799,10.1190258596251,4.97344565700631));
#10736=CARTESIAN_POINT('Ctrl Pts',(-3.8030697228604,11.0693349098104,5.64394863077188));
#10737=CARTESIAN_POINT('Ctrl Pts',(-2.92780373849181,11.3212163217078,5.8639559865285));
#10738=CARTESIAN_POINT('Ctrl Pts',(-2.04522493875568,11.4685794314074,6.04489666046755));
#10739=CARTESIAN_POINT('',(-10.9838133703314,3.97811209444304,8.08507411790788));
#10740=CARTESIAN_POINT('Ctrl Pts',(-11.0841054060657,3.97811209444304,2.68507522891397));
#10741=CARTESIAN_POINT('Ctrl Pts',(-11.0671368467592,3.97811209444304,3.59910749288785));
#10742=CARTESIAN_POINT('Ctrl Pts',(-11.0501656900449,3.97811209444304,4.51314082004822));
#10743=CARTESIAN_POINT('Ctrl Pts',(-11.0331899258266,3.97811209444304,5.42717406162499));
#10744=CARTESIAN_POINT('Ctrl Pts',(-11.0167354225938,3.97811209444304,6.31314082783784));
#10745=CARTESIAN_POINT('Ctrl Pts',(-11.0002765904705,3.97811209444304,7.1991075136423));
#10746=CARTESIAN_POINT('Ctrl Pts',(-10.9838133703314,3.97811209444304,8.08507411790788));
#10747=CARTESIAN_POINT('',(-11.6873575570212,1.20571420530696E-6,8.08507411790788));
#10748=CARTESIAN_POINT('Origin',(-0.0886968229780924,1.20571420388653E-6,
8.08507411790788));
#10749=CARTESIAN_POINT('',(-11.2742087842189,1.20571420492242E-6,31.7543514595497));
#10750=CARTESIAN_POINT('',(-11.7886968229781,1.20571420531937E-6,2.2793514595497));
#10751=CARTESIAN_POINT('',(11.096827150046,1.20571420194828E-6,31.7536633049461));
#10752=CARTESIAN_POINT('Ctrl Pts',(-11.2742087842189,1.20571420458848E-6,
31.7543514595497));
#10753=CARTESIAN_POINT('Ctrl Pts',(-11.2742087842189,0.714879232030262,
31.7543514595497));
#10754=CARTESIAN_POINT('Ctrl Pts',(-11.2039243099315,1.44919356167399,31.793099916814));
#10755=CARTESIAN_POINT('Ctrl Pts',(-10.9133728006453,2.90079942562337,31.9472948843815));
#10756=CARTESIAN_POINT('Ctrl Pts',(-10.6932214582039,3.61814006950708,32.0624969509637));
#10757=CARTESIAN_POINT('Ctrl Pts',(-9.82880176569562,5.67152012999344,32.4870523054472));
#10758=CARTESIAN_POINT('Ctrl Pts',(-8.96991780652531,6.90812806220324,32.8751111589287));
#10759=CARTESIAN_POINT('Ctrl Pts',(-7.00675772315132,8.85727351788031,33.5789580196972));
#10760=CARTESIAN_POINT('Ctrl Pts',(-5.76477228566963,9.70843557232902,33.9447939157601));
#10761=CARTESIAN_POINT('Ctrl Pts',(-3.01891541115682,10.8482984598267,34.4584272670688));
#10762=CARTESIAN_POINT('Ctrl Pts',(-1.51351007601002,11.1358317415463,34.6005984149743));
#10763=CARTESIAN_POINT('Ctrl Pts',(1.33613242402791,11.1358330727219,34.6005221519735));
#10764=CARTESIAN_POINT('Ctrl Pts',(2.84154593721425,10.8482953636761,34.4582674767084));
#10765=CARTESIAN_POINT('Ctrl Pts',(5.58740871904998,9.70842501571461,33.9444749141113));
#10766=CARTESIAN_POINT('Ctrl Pts',(6.82939227785914,8.85726022067858,33.578563036809));
#10767=CARTESIAN_POINT('Ctrl Pts',(8.79254166028598,6.90811816343161,32.8745913568126));
#10768=CARTESIAN_POINT('Ctrl Pts',(9.65142087432493,5.67151703383353,32.4864738899089));
#10769=CARTESIAN_POINT('Ctrl Pts',(10.5158385377037,3.61814283629084,32.0618549656255));
#10770=CARTESIAN_POINT('Ctrl Pts',(10.7359899995928,2.90080333450706,31.9466357770987));
#10771=CARTESIAN_POINT('Ctrl Pts',(11.0265421577798,1.44919736945254,31.7924176982799));
#10772=CARTESIAN_POINT('Ctrl Pts',(11.096827150046,0.714881784716172,31.7536633049461));
#10773=CARTESIAN_POINT('Ctrl Pts',(11.096827150046,1.20571420431093E-6,
31.7536633049461));
#10774=CARTESIAN_POINT('Ctrl Pts',(11.096827150046,1.20571420389459E-6,
31.7536633049461));
#10775=CARTESIAN_POINT('Ctrl Pts',(11.096827150046,-0.714879373287764,31.7536633049461));
#10776=CARTESIAN_POINT('Ctrl Pts',(11.0265421577798,-1.44919495802413,31.7924176982799));
#10777=CARTESIAN_POINT('Ctrl Pts',(10.7359899995928,-2.90080092307865,31.9466357770987));
#10778=CARTESIAN_POINT('Ctrl Pts',(10.5158385377037,-3.61814042486243,32.0618549656255));
#10779=CARTESIAN_POINT('Ctrl Pts',(9.65142087432494,-5.67151462240512,32.4864738899089));
#10780=CARTESIAN_POINT('Ctrl Pts',(8.79254166028598,-6.9081157520032,32.8745913568126));
#10781=CARTESIAN_POINT('Ctrl Pts',(6.82939227785914,-8.85725780925017,33.578563036809));
#10782=CARTESIAN_POINT('Ctrl Pts',(5.58740871904998,-9.70842260428621,33.9444749141113));
#10783=CARTESIAN_POINT('Ctrl Pts',(2.84154593721424,-10.8482929522477,34.4582674767085));
#10784=CARTESIAN_POINT('Ctrl Pts',(1.33613242402791,-11.1358306612935,34.6005221519735));
#10785=CARTESIAN_POINT('Ctrl Pts',(-1.51351007601001,-11.1358293301179,
34.6005984149743));
#10786=CARTESIAN_POINT('Ctrl Pts',(-3.01891541115682,-10.8482960483983,
34.4584272670688));
#10787=CARTESIAN_POINT('Ctrl Pts',(-5.76477228566962,-9.70843316090061,
33.9447939157601));
#10788=CARTESIAN_POINT('Ctrl Pts',(-7.00675772315132,-8.85727110645191,
33.5789580196972));
#10789=CARTESIAN_POINT('Ctrl Pts',(-8.96991780652531,-6.90812565077484,
32.8751111589287));
#10790=CARTESIAN_POINT('Ctrl Pts',(-9.82880176569561,-5.67151771856503,
32.4870523054472));
#10791=CARTESIAN_POINT('Ctrl Pts',(-10.6932214582039,-3.61813765807868,
32.0624969509637));
#10792=CARTESIAN_POINT('Ctrl Pts',(-10.9133728006453,-2.90079701419497,
31.9472948843814));
#10793=CARTESIAN_POINT('Ctrl Pts',(-11.2039243099315,-1.44919115024558,
31.793099916814));
#10794=CARTESIAN_POINT('Ctrl Pts',(-11.2742087842189,-0.714876820601855,
31.7543514595497));
#10795=CARTESIAN_POINT('Ctrl Pts',(-11.2742087842189,1.20571420417215E-6,
31.7543514595497));
#10796=CARTESIAN_POINT('',(-10.9838133703314,-3.97810968301463,8.08507411790788));
#10797=CARTESIAN_POINT('Origin',(-0.0886968229780924,1.20571420388653E-6,
8.08507411790788));
#10798=CARTESIAN_POINT('',(-11.084104180594,-3.97810913882278,2.68507514951319));
#10799=CARTESIAN_POINT('Ctrl Pts',(-10.9838133703314,-3.97810968301463,
8.08507411790788));
#10800=CARTESIAN_POINT('Ctrl Pts',(-11.0002765904705,-3.97810968301463,
7.19910751364231));
#10801=CARTESIAN_POINT('Ctrl Pts',(-11.016735422596,-3.97810968301463,6.31314082782715));
#10802=CARTESIAN_POINT('Ctrl Pts',(-11.0331899258289,-3.97810968301463,
5.42717406161412));
#10803=CARTESIAN_POINT('Ctrl Pts',(-11.0501656900472,-3.97810968301463,
4.51314082003718));
#10804=CARTESIAN_POINT('Ctrl Pts',(-11.0671368467592,-3.97810968301463,
3.59910749288785));
#10805=CARTESIAN_POINT('Ctrl Pts',(-11.0841054060657,-3.97810968301463,
2.68507522891397));
#10806=CARTESIAN_POINT('',(-2.04522493875568,-11.468577019979,6.04489666046755));
#10807=CARTESIAN_POINT('Ctrl Pts',(-2.04522493875568,-11.468577019979,6.04489666046755));
#10808=CARTESIAN_POINT('Ctrl Pts',(-2.92780373849181,-11.3212139102794,
5.8639559865285));
#10809=CARTESIAN_POINT('Ctrl Pts',(-3.8030697228604,-11.069332498382,5.64394863077188));
#10810=CARTESIAN_POINT('Ctrl Pts',(-6.07582291747798,-10.1190234481967,
4.97344565700631));
#10811=CARTESIAN_POINT('Ctrl Pts',(-7.3782638345928,-9.21886015324496,4.47105415851212));
#10812=CARTESIAN_POINT('Ctrl Pts',(-9.4105044355921,-7.17555942422152,3.57669501792372));
#10813=CARTESIAN_POINT('Ctrl Pts',(-10.2946364808206,-5.89560114630819,
3.11981222038324));
#10814=CARTESIAN_POINT('Ctrl Pts',(-10.9580372989578,-4.31099264715397,
2.75525104909032));
#10815=CARTESIAN_POINT('Ctrl Pts',(-11.0229709537136,-4.14532589001081,
2.71923525419232));
#10816=CARTESIAN_POINT('Ctrl Pts',(-11.0841037493982,-3.97810877586148,
2.68507615460814));
#10817=CARTESIAN_POINT('',(3.79009320173104,-10.9020986117265,9.63818989051917));
#10818=CARTESIAN_POINT('Ctrl Pts',(-2.04522493875568,-11.468577019979,6.04489666046755));
#10819=CARTESIAN_POINT('Ctrl Pts',(-1.32470976378382,-11.5888805631882,
6.19261208415742));
#10820=CARTESIAN_POINT('Ctrl Pts',(-0.617178694535787,-11.6334191099327,
6.42377887019057));
#10821=CARTESIAN_POINT('Ctrl Pts',(0.581234136539686,-11.6122832538287,
6.95921219643471));
#10822=CARTESIAN_POINT('Ctrl Pts',(1.16082935689865,-11.5580643111816,7.28307730157583));
#10823=CARTESIAN_POINT('Ctrl Pts',(2.23455214075372,-11.3774703929902,8.03794303289295));
#10824=CARTESIAN_POINT('Ctrl Pts',(2.72899476230882,-11.2526075426344,8.46885648760705));
#10825=CARTESIAN_POINT('Ctrl Pts',(3.36708944887808,-11.055272086373,9.13007814566771));
#10826=CARTESIAN_POINT('Ctrl Pts',(3.58403350493311,-10.9802387496915,9.37762586958811));
#10827=CARTESIAN_POINT('Ctrl Pts',(3.79009320173103,-10.9020986117265,9.63818989051917));
#10828=CARTESIAN_POINT('',(9.21661950459473,-6.7499987942858,13.9829593621724));
#10829=CARTESIAN_POINT('Ctrl Pts',(9.21661950459473,-6.74999879428579,13.9829593621724));
#10830=CARTESIAN_POINT('Ctrl Pts',(9.0022731985786,-7.04855619626984,13.8797875988384));
#10831=CARTESIAN_POINT('Ctrl Pts',(8.77823970806681,-7.33062270822828,13.765805640045));
#10832=CARTESIAN_POINT('Ctrl Pts',(8.04927182637234,-8.17020632231756,13.3703563763539));
#10833=CARTESIAN_POINT('Ctrl Pts',(7.45983969473753,-8.72586176044201,13.0128149073975));
#10834=CARTESIAN_POINT('Ctrl Pts',(6.25376498977623,-9.65635517599508,12.1401590568172));
#10835=CARTESIAN_POINT('Ctrl Pts',(5.63962932833512,-10.0329229670701,11.623427806388));
#10836=CARTESIAN_POINT('Ctrl Pts',(4.64694412836354,-10.5510419920863,10.650798216911));
#10837=CARTESIAN_POINT('Ctrl Pts',(4.20613537995868,-10.7443307720609,10.1642783227575));
#10838=CARTESIAN_POINT('Ctrl Pts',(3.79009320173104,-10.9020986117265,9.63818989051917));
#10839=CARTESIAN_POINT('Ctrl Pts',(9.15430644803649,-6.7499987942858,16.869309255546));
#10840=CARTESIAN_POINT('Ctrl Pts',(9.17510170146438,-6.7499987942858,15.9071931479241));
#10841=CARTESIAN_POINT('Ctrl Pts',(9.19587255806942,-6.7499987942858,14.9450765126902));
#10842=CARTESIAN_POINT('Ctrl Pts',(9.21661950459473,-6.7499987942858,13.9829593621724));
#10843=CARTESIAN_POINT('Origin',(4.28112241113661,32.4000012057142,-24.8132842517073));
#10844=CARTESIAN_POINT('',(-7.28869682297809,-6.7499987942858,4.48499697586492));
#10845=CARTESIAN_POINT('',(-2.04522493875568,-6.7499987942858,6.04489666046755));
#10846=CARTESIAN_POINT('Origin',(4.28112241113661,-6.7499987942858,-24.8132842517073));
#10847=CARTESIAN_POINT('',(-2.04522493875568,32.4000012057142,6.04489666046755));
#10848=CARTESIAN_POINT('Ctrl Pts',(-11.0841037493982,-3.97810877586148,
2.68507615460814));
#10849=CARTESIAN_POINT('Ctrl Pts',(-11.2880488632369,-3.42025577733562,
2.57111798575136));
#10850=CARTESIAN_POINT('Ctrl Pts',(-11.4494008749826,-2.8449890145717,2.47808040767037));
#10851=CARTESIAN_POINT('Ctrl Pts',(-11.7156745135564,-1.50931079877612,
2.32309001764736));
#10852=CARTESIAN_POINT('Ctrl Pts',(-11.7886968229781,-0.744842394221963,
2.2793514595497));
#10853=CARTESIAN_POINT('Ctrl Pts',(-11.7886968229781,0.744844805650374,
2.2793514595497));
#10854=CARTESIAN_POINT('Ctrl Pts',(-11.7156745135564,1.50931321020453,2.32309001764737));
#10855=CARTESIAN_POINT('Ctrl Pts',(-11.4494008749826,2.84499142600011,2.47808040767037));
#10856=CARTESIAN_POINT('Ctrl Pts',(-11.2880488632369,3.42025818876404,2.57111798575136));
#10857=CARTESIAN_POINT('Ctrl Pts',(-11.0841037493982,3.97811118728989,2.68507615460815));
#10858=CARTESIAN_POINT('',(-2.04522493875568,6.7500012057142,6.04489666046755));
#10859=CARTESIAN_POINT('',(-2.04522493875568,32.4000012057142,6.04489666046755));
#10860=CARTESIAN_POINT('',(-7.28869682297809,6.7500012057142,4.48499697586491));
#10861=CARTESIAN_POINT('Origin',(4.28112241113661,6.75000120571421,-24.8132842517073));
#10862=CARTESIAN_POINT('',(-7.28869682297809,32.4000012057142,4.48499697586492));
#10863=CARTESIAN_POINT('Origin',(-10.1906081922044,1.20571420388653E-6,
-7.82255990967661));
#10864=CARTESIAN_POINT('',(-16.8798656013815,-3.97810968301463,-1.13330250049948));
#10865=CARTESIAN_POINT('',(-18.3070733952457,-3.97810968301463,0.293905293364732));
#10866=CARTESIAN_POINT('',(-16.2434694983136,-3.97810968301463,-1.76969860356737));
#10867=CARTESIAN_POINT('',(-18.3070733952457,-2.2499987942858,0.293905293364733));
#10868=CARTESIAN_POINT('',(-18.3070733952457,-2.2499987942858,0.293905293364733));
#10869=CARTESIAN_POINT('',(-16.8798656013815,-2.2499987942858,-1.13330250049948));
#10870=CARTESIAN_POINT('',(-10.1906081922044,-2.2499987942858,-7.82255990967661));
#10871=CARTESIAN_POINT('',(-16.8798656013815,-3.97810968301463,-1.13330250049948));
#10872=CARTESIAN_POINT('Origin',(-0.0886968229780924,1.20571420388653E-6,
2.2793514595497));
#10873=CARTESIAN_POINT('Origin',(-0.0886968229780924,1.20571420388653E-6,
2.68507411790788));
#10874=CARTESIAN_POINT('Origin',(-0.0893230609073105,32.4000012057142,11.2005602920677));
#10875=CARTESIAN_POINT('',(6.61050363813806,-3.97810968301463,33.6209153785234));
#10876=CARTESIAN_POINT('',(6.61050363813806,3.97811209444304,33.6209153785234));
#10877=CARTESIAN_POINT('',(6.61050363813806,32.4000012057142,33.6209153785234));
#10878=CARTESIAN_POINT('',(-6.78789728409425,-3.97810968301463,33.621289615095));
#10879=CARTESIAN_POINT('Origin',(-0.0893230609073105,-3.97810968301463,
11.2005602920677));
#10880=CARTESIAN_POINT('',(-6.78789728409425,3.97811209444304,33.621289615095));
#10881=CARTESIAN_POINT('',(-6.78789728409425,32.4000012057142,33.621289615095));
#10882=CARTESIAN_POINT('Origin',(-0.0893230609073105,3.97811209444304,11.2005602920677));
#10883=CARTESIAN_POINT('Origin',(14.3113031770219,6.7500012057142,14.8344044426714));
#10884=CARTESIAN_POINT('',(6.51868832412356,6.7500012057142,14.8344044426714));
#10885=CARTESIAN_POINT('',(6.51868832412356,-6.7499987942858,14.8344044426714));
#10886=CARTESIAN_POINT('Origin',(-0.0886968229780924,1.20571420076229E-6,
14.8344044426714));
#10887=CARTESIAN_POINT('',(-7.28869682297809,-6.7499987942858,14.8344044426714));
#10888=CARTESIAN_POINT('',(14.3113031770219,-6.7499987942858,14.8344044426714));
#10889=CARTESIAN_POINT('',(-7.28869682297809,6.7500012057142,14.8344044426714));
#10890=CARTESIAN_POINT('',(-7.28869682297809,6.7500012057142,14.8344044426714));
#10891=CARTESIAN_POINT('',(14.3113031770219,6.7500012057142,14.8344044426714));
#10892=CARTESIAN_POINT('Origin',(14.3113031770219,-6.7499987942858,-10.275701523572));
#10893=CARTESIAN_POINT('',(3.79009320173104,-6.74999879428579,9.63818989051917));
#10894=CARTESIAN_POINT('Origin',(15.9282673556341,-6.74999879428579,0.0390576814896602));
#10895=CARTESIAN_POINT('Origin',(-4.05358917681673,-6.7499987942858,15.8411445690945));
#10896=CARTESIAN_POINT('',(-7.28869682297809,-6.7499987942858,-10.275701523572));
#10897=CARTESIAN_POINT('Ctrl Pts',(6.51868832412356,-6.7499987942858,14.8344044426714));
#10898=CARTESIAN_POINT('Ctrl Pts',(6.89318504201329,-6.7499987942858,14.8344044426714));
#10899=CARTESIAN_POINT('Ctrl Pts',(7.33776310853797,-6.7499987942858,14.9000334212391));
#10900=CARTESIAN_POINT('Ctrl Pts',(7.97286532132927,-6.7499987942858,15.1264890486251));
#10901=CARTESIAN_POINT('Ctrl Pts',(8.28752674897206,-6.7499987942858,15.3008175202491));
#10902=CARTESIAN_POINT('Ctrl Pts',(8.70384046495954,-6.7499987942858,15.665664492641));
#10903=CARTESIAN_POINT('Ctrl Pts',(8.89134878165894,-6.7499987942858,15.9056447643772));
#10904=CARTESIAN_POINT('Ctrl Pts',(9.09386350816702,-6.7499987942858,16.3417623265294));
#10905=CARTESIAN_POINT('Ctrl Pts',(9.15468363432064,-6.7499987942858,16.6073512291574));
#10906=CARTESIAN_POINT('Ctrl Pts',(9.15468363432064,-6.7499987942858,16.8344044426714));
#10907=CARTESIAN_POINT('Ctrl Pts',(9.15468363432064,-6.7499987942858,16.8459433493969));
#10908=CARTESIAN_POINT('Ctrl Pts',(9.15455990443804,-6.7499987942858,16.8575828061736));
#10909=CARTESIAN_POINT('Ctrl Pts',(9.15430644803649,-6.7499987942858,16.869309255546));
#10910=CARTESIAN_POINT('Origin',(14.3113031770219,6.7500012057142,-10.275701523572));
#10911=CARTESIAN_POINT('',(3.79009320173104,6.7500012057142,9.63818989051917));
#10912=CARTESIAN_POINT('Origin',(-4.05358917681673,6.7500012057142,15.8411445690945));
#10913=CARTESIAN_POINT('Origin',(15.9282673556341,6.7500012057142,0.0390576814896602));
#10914=CARTESIAN_POINT('Ctrl Pts',(9.15430644803649,6.7500012057142,16.8693092555461));
#10915=CARTESIAN_POINT('Ctrl Pts',(9.1545597299,6.7500012057142,16.8575908813751));
#10916=CARTESIAN_POINT('Ctrl Pts',(9.15468363432064,6.7500012057142,16.8459519530649));
#10917=CARTESIAN_POINT('Ctrl Pts',(9.15468363432064,6.7500012057142,16.8344044426714));
#10918=CARTESIAN_POINT('Ctrl Pts',(9.15468363432064,6.7500012057142,16.6073512291574));
#10919=CARTESIAN_POINT('Ctrl Pts',(9.09386350816702,6.7500012057142,16.3417623265294));
#10920=CARTESIAN_POINT('Ctrl Pts',(8.89134878165894,6.7500012057142,15.9056447643772));
#10921=CARTESIAN_POINT('Ctrl Pts',(8.70384046495954,6.7500012057142,15.665664492641));
#10922=CARTESIAN_POINT('Ctrl Pts',(8.28752674897205,6.7500012057142,15.3008175202491));
#10923=CARTESIAN_POINT('Ctrl Pts',(7.97286532132927,6.7500012057142,15.126489048625));
#10924=CARTESIAN_POINT('Ctrl Pts',(7.33776310853796,6.7500012057142,14.9000334212391));
#10925=CARTESIAN_POINT('Ctrl Pts',(6.89318504201329,6.7500012057142,14.8344044426714));
#10926=CARTESIAN_POINT('Ctrl Pts',(6.51868832412356,6.7500012057142,14.8344044426714));
#10927=CARTESIAN_POINT('',(-7.28869682297809,6.7500012057142,-10.275701523572));
#10928=CARTESIAN_POINT('Origin',(-7.28869682297809,1.20571420388653E-6,
2.2793514595497));
#10929=CARTESIAN_POINT('Origin',(11.8416209672313,-3.97810968301463,2.68507411790788));
#10930=CARTESIAN_POINT('',(-11.7886967768384,-3.97810968301463,2.68507411790788));
#10931=CARTESIAN_POINT('',(11.8416209672313,-3.97810968301463,2.68507411790788));
#10932=CARTESIAN_POINT('',(-11.7886967768384,3.97811209444304,2.68507411790788));
#10933=CARTESIAN_POINT('',(-11.7886967768384,-3.97810968301463,2.68507411790788));
#10934=CARTESIAN_POINT('',(11.8416209672313,3.97811209444304,2.68507411790788));
#10935=CARTESIAN_POINT('Origin',(11.8416209672313,3.97811209444304,8.08507411790788));
#10936=CARTESIAN_POINT('',(-18.3070733952457,3.97811209444304,0.293905293364732));
#10937=CARTESIAN_POINT('',(-16.8798656013815,3.97811209444304,-1.13330250049948));
#10938=CARTESIAN_POINT('',(-18.9434694983136,3.97811209444304,0.930301396432627));
#10939=CARTESIAN_POINT('',(-18.3070733952457,3.97811209444304,1.56669749950052));
#10940=CARTESIAN_POINT('Origin',(-17.6706772921778,3.97811209444304,0.930301396432626));
#10941=CARTESIAN_POINT('',(-11.7886967768384,3.97811209444304,8.08507411790788));
#10942=CARTESIAN_POINT('',(-18.9434694983136,3.97811209444304,0.930301396432627));
#10943=CARTESIAN_POINT('',(11.8416209672313,3.97811209444304,8.08507411790788));
#10944=CARTESIAN_POINT('',(-15.6070733952457,3.97811209444304,-1.13330250049948));
#10945=CARTESIAN_POINT('',(-16.2434694983136,3.97811209444304,-1.76969860356737));
#10946=CARTESIAN_POINT('Origin',(-16.2434694983136,3.97811209444304,-0.496906397431586));
#10947=CARTESIAN_POINT('Origin',(11.8416209672313,-3.97810968301463,8.08507411790788));
#10948=CARTESIAN_POINT('',(-11.7886967768384,-3.97810968301463,8.08507411790788));
#10949=CARTESIAN_POINT('',(-11.7886967768384,-3.97810968301463,8.08507411790788));
#10950=CARTESIAN_POINT('',(11.8416209672313,-3.97810968301463,8.08507411790788));
#10951=CARTESIAN_POINT('Origin',(11.8416209672313,-3.97810968301463,8.08507411790788));
#10952=CARTESIAN_POINT('',(-18.3070733952457,-3.97810968301463,1.56669749950052));
#10953=CARTESIAN_POINT('',(-18.9434694983136,-3.97810968301463,0.930301396432627));
#10954=CARTESIAN_POINT('Origin',(-17.6706772921778,-3.97810968301463,0.930301396432626));
#10955=CARTESIAN_POINT('',(-15.6070733952457,-3.97810968301463,-1.13330250049948));
#10956=CARTESIAN_POINT('Origin',(-16.2434694983136,-3.97810968301463,-0.496906397431586));
#10957=CARTESIAN_POINT('',(-16.2434694983136,-3.97810968301463,-1.76969860356737));
#10958=CARTESIAN_POINT('Origin',(-16.2434694983136,3.97811209444304,-1.76969860356737));
#10959=CARTESIAN_POINT('',(-15.6070733952457,-2.2499987942858,-1.13330250049948));
#10960=CARTESIAN_POINT('',(-15.6070733952457,-2.2499987942858,-1.13330250049948));
#10961=CARTESIAN_POINT('',(-12.4250928799063,-2.2499987942858,2.04867801483998));
#10962=CARTESIAN_POINT('',(-16.2434694983136,-2.2499987942858,-1.76969860356737));
#10963=CARTESIAN_POINT('',(-12.4250928799063,2.2500012057142,2.04867801483998));
#10964=CARTESIAN_POINT('',(-12.4250928799063,3.97811209444304,2.04867801483998));
#10965=CARTESIAN_POINT('',(-15.6070733952457,2.2500012057142,-1.13330250049948));
#10966=CARTESIAN_POINT('',(-16.2434694983136,2.2500012057142,-1.76969860356737));
#10967=CARTESIAN_POINT('',(-15.6070733952457,3.97811209444304,-1.13330250049948));
#10968=CARTESIAN_POINT('Origin',(-18.9434694983136,-3.97810968301463,0.930301396432627));
#10969=CARTESIAN_POINT('',(-15.1250928799063,2.2500012057142,4.74867801483998));
#10970=CARTESIAN_POINT('',(-18.3070733952457,2.2500012057142,1.56669749950052));
#10971=CARTESIAN_POINT('',(-22.1254500136531,2.2500012057142,-2.25167911890684));
#10972=CARTESIAN_POINT('',(-15.1250928799063,-2.2499987942858,4.74867801483998));
#10973=CARTESIAN_POINT('',(-15.1250928799063,-3.97810968301463,4.74867801483998));
#10974=CARTESIAN_POINT('',(-18.3070733952457,-2.2499987942858,1.56669749950052));
#10975=CARTESIAN_POINT('',(-22.1254500136531,-2.2499987942858,-2.25167911890684));
#10976=CARTESIAN_POINT('',(-18.3070733952457,-3.97810968301463,1.56669749950052));
#10977=CARTESIAN_POINT('',(-18.3070733952457,2.2500012057142,1.56669749950052));
#10978=CARTESIAN_POINT('Origin',(-10.1906081922044,1.20571420388653E-6,
-7.82255990967661));
#10979=CARTESIAN_POINT('',(-18.3070733952457,2.2500012057142,0.293905293364733));
#10980=CARTESIAN_POINT('',(-16.8798656013815,2.2500012057142,-1.13330250049948));
#10981=CARTESIAN_POINT('',(-10.1906081922044,2.2500012057142,-7.82255990967661));
#10982=CARTESIAN_POINT('',(-18.3070733952457,3.97811209444304,0.293905293364733));
#10983=CARTESIAN_POINT('',(-16.8798656013815,2.2500012057142,-1.13330250049948));
#10984=CARTESIAN_POINT('Origin',(-11.3067162614989,2.2500012057142,-0.342490809703158));
#10985=CARTESIAN_POINT('',(-13.6978850860421,-2.2499987942858,2.04867801483998));
#10986=CARTESIAN_POINT('',(-15.1250928799063,-2.2499987942858,3.4758858087042));
#10987=CARTESIAN_POINT('',(-11.3067162614989,-2.2499987942858,-0.342490809703158));
#10988=CARTESIAN_POINT('',(-15.1250928799063,2.2500012057142,3.4758858087042));
#10989=CARTESIAN_POINT('',(-15.1250928799063,2.2500012057142,3.4758858087042));
#10990=CARTESIAN_POINT('',(-13.6978850860421,2.2500012057142,2.04867801483998));
#10991=CARTESIAN_POINT('',(-11.3067162614989,2.2500012057142,-0.342490809703158));
#10992=CARTESIAN_POINT('',(-13.6978850860421,2.2500012057142,2.04867801483998));
#10993=CARTESIAN_POINT('Origin',(-17.6706772921778,-2.2499987942858,-6.70645184038209));
#10994=CARTESIAN_POINT('Origin',(-17.6706772921778,-2.2499987942858,0.930301396432626));
#10995=CARTESIAN_POINT('Origin',(-14.4886967768384,-2.2499987942858,4.11228191177209));
#10996=CARTESIAN_POINT('Origin',(-13.0614889829742,-2.2499987942858,2.68507411790788));
#10997=CARTESIAN_POINT('Origin',(-16.2434694983136,-2.2499987942858,-0.496906397431586));
#10998=CARTESIAN_POINT('Origin',(-17.6706772921778,2.2500012057142,-6.70645184038209));
#10999=CARTESIAN_POINT('Origin',(-17.6706772921778,2.2500012057142,0.930301396432626));
#11000=CARTESIAN_POINT('Origin',(-16.2434694983136,2.2500012057142,-0.496906397431586));
#11001=CARTESIAN_POINT('Origin',(-13.0614889829742,2.2500012057142,2.68507411790788));
#11002=CARTESIAN_POINT('Origin',(-14.4886967768384,2.2500012057142,4.11228191177209));
#11003=CARTESIAN_POINT('Origin',(-16.3206772921779,-4.87810968301463,0.853093602568413));
#11004=CARTESIAN_POINT('Origin',(-16.3206772921779,4.87789031698537,0.853093602568413));
#11005=CARTESIAN_POINT('Origin',(-14.4886967768384,2.2500012057142,4.11228191177209));
#11006=CARTESIAN_POINT('Origin',(-17.6706772921778,1.20571420388653E-6,
0.930301396432626));
#11007=CARTESIAN_POINT('Origin',(-17.6706772921778,1.20571420388653E-6,
0.930301396432626));
#11008=CARTESIAN_POINT('Origin',(-16.2434694983136,1.20571420388653E-6,
-0.496906397431586));
#11009=CARTESIAN_POINT('Origin',(-16.2434694983136,1.20571420388653E-6,
-0.496906397431586));
#11010=CARTESIAN_POINT('Origin',(-13.0614889829742,3.97811209444304,2.68507411790788));
#11011=CARTESIAN_POINT('Origin',(-0.0886968229780924,1.20571420388653E-6,
42.7793514595497));
#11012=CARTESIAN_POINT('',(-4.08789728409425,-3.97810968301463,42.7793514595497));
#11013=CARTESIAN_POINT('',(3.91050363813806,-3.97810968301463,42.7793514595497));
#11014=CARTESIAN_POINT('',(6.61050363813806,-3.97810968301463,42.7793514595497));
#11015=CARTESIAN_POINT('',(3.91050363813806,3.97811209444304,42.7793514595497));
#11016=CARTESIAN_POINT('',(3.91050363813806,3.97811209444304,42.7793514595497));
#11017=CARTESIAN_POINT('',(-4.08789728409425,3.97811209444304,42.7793514595497));
#11018=CARTESIAN_POINT('',(6.61050363813806,3.97811209444304,42.7793514595497));
#11019=CARTESIAN_POINT('',(-4.08789728409424,-3.97810968301463,42.7793514595497));
#11020=CARTESIAN_POINT('Origin',(6.61050363813806,-3.97810968301463,-1.39780639743159));
#11021=CARTESIAN_POINT('',(6.61050363813806,-3.97810968301463,40.0793514595497));
#11022=CARTESIAN_POINT('',(6.61050363813806,-3.97810968301463,-1.39780639743159));
#11023=CARTESIAN_POINT('Origin',(3.91050363813806,-3.97810968301463,40.0793514595497));
#11024=CARTESIAN_POINT('',(-6.78789728409425,-3.97810968301463,40.0793514595497));
#11025=CARTESIAN_POINT('Origin',(-4.08789728409424,-3.97810968301463,40.0793514595497));
#11026=CARTESIAN_POINT('',(-6.78789728409425,-3.97810968301463,-1.39780639743159));
#11027=CARTESIAN_POINT('Origin',(6.61050363813806,3.97811209444304,-1.39780639743159));
#11028=CARTESIAN_POINT('',(6.61050363813806,3.97811209444304,40.0793514595497));
#11029=CARTESIAN_POINT('',(6.61050363813806,3.97811209444304,-1.39780639743159));
#11030=CARTESIAN_POINT('',(6.61050363813806,-3.97810968301463,40.0793514595497));
#11031=CARTESIAN_POINT('Origin',(6.61050363813806,3.97811209444304,-1.39780639743159));
#11032=CARTESIAN_POINT('Origin',(3.91050363813806,3.97811209444304,40.0793514595497));
#11033=CARTESIAN_POINT('',(-6.78789728409425,3.97811209444304,40.0793514595497));
#11034=CARTESIAN_POINT('',(-6.78789728409425,3.97811209444304,-1.39780639743159));
#11035=CARTESIAN_POINT('Origin',(-4.08789728409424,3.97811209444304,40.0793514595497));
#11036=CARTESIAN_POINT('Origin',(-6.78789728409425,3.97811209444304,-1.39780639743159));
#11037=CARTESIAN_POINT('',(-6.78789728409425,3.97811209444304,40.0793514595497));
#11038=CARTESIAN_POINT('Origin',(3.91050363813806,1.20571420388653E-6,40.0793514595497));
#11039=CARTESIAN_POINT('Origin',(-4.08789728409424,1.20571420388653E-6,
40.0793514595497));
#11040=CARTESIAN_POINT('Origin',(15.9282673556341,20.,0.0390576814896602));
#11041=CARTESIAN_POINT('',(3.79009320173104,20.,9.63818989051917));
#11042=CARTESIAN_POINT('Origin',(15.9282673556341,20.,0.0390576814896602));
#11043=CARTESIAN_POINT('',(3.79009320173104,20.,9.63818989051917));
#11044=CARTESIAN_POINT('Origin',(-4.05358917681673,20.,15.8411445690945));
#11045=CARTESIAN_POINT('Origin',(-4.05358917681673,20.,15.8411445690945));
#11046=CARTESIAN_POINT('Origin',(-0.0886968229780924,1.205714200531E-6,
16.8344044426714));
#13152=UNCERTAINTY_MEASURE_WITH_UNIT(LENGTH_MEASURE(0.01),#13200,
'DISTANCE_ACCURACY_VALUE',
'Maximum model space distance between geometric entities at asserted c
onnectivities');
#13173=UNCERTAINTY_MEASURE_WITH_UNIT(LENGTH_MEASURE(0.01),#13200,
'DISTANCE_ACCURACY_VALUE',
'Maximum model space distance between geometric entities at asserted c
onnectivities');
#13178=(
GEOMETRIC_REPRESENTATION_CONTEXT(3)
GLOBAL_UNCERTAINTY_ASSIGNED_CONTEXT((#13152))
GLOBAL_UNIT_ASSIGNED_CONTEXT((#13200,#13202,#13203))
REPRESENTATION_CONTEXT('','3D')
);
#13199=(
GEOMETRIC_REPRESENTATION_CONTEXT(3)
GLOBAL_UNCERTAINTY_ASSIGNED_CONTEXT((#13173))
GLOBAL_UNIT_ASSIGNED_CONTEXT((#13200,#13202,#13203))
REPRESENTATION_CONTEXT('','3D')
);
#13200=(
LENGTH_UNIT()
NAMED_UNIT(*)
SI_UNIT(.MILLI.,.METRE.)
);
#13202=(
NAMED_UNIT(*)
PLANE_ANGLE_UNIT()
SI_UNIT($,.RADIAN.)
);
#13203=(
NAMED_UNIT(*)
SI_UNIT($,.STERADIAN.)
SOLID_ANGLE_UNIT()
);
#13208=SHAPE_DEFINITION_REPRESENTATION(#13233,#13282);
#13233=PRODUCT_DEFINITION_SHAPE('',$,#13308);
#13282=SHAPE_REPRESENTATION('',(#7274),#13178);
#13303=PRODUCT_DEFINITION_CONTEXT('part definition',#13380,'design');
#13308=PRODUCT_DEFINITION('Finger Link 2','Finger Link 2',#13333,#13303);
#13333=PRODUCT_DEFINITION_FORMATION('',$,#13386);
#13380=APPLICATION_CONTEXT(
'Core Data for Automotive Mechanical Design Process');
#13381=PRODUCT_CONTEXT('part definition',#13380,'mechanical');
#13386=PRODUCT('Finger Link 2','Finger Link 2',$,(#13381));
#13409=PRESENTATION_STYLE_ASSIGNMENT((#13414));
#13414=SURFACE_STYLE_USAGE(.BOTH.,#13419);
#13419=SURFACE_SIDE_STYLE('',(#13424));
#13424=SURFACE_STYLE_FILL_AREA(#13429);
#13429=FILL_AREA_STYLE('Opaque(61,176,222)',(#13434));
#13434=FILL_AREA_STYLE_COLOUR('Opaque(61,176,222)',#13439);
#13439=COLOUR_RGB('Opaque(61,176,222)',0.23921568627451,0.690196078431373,
0.870588235294118);
ENDSEC;
END-ISO-10303-21;
